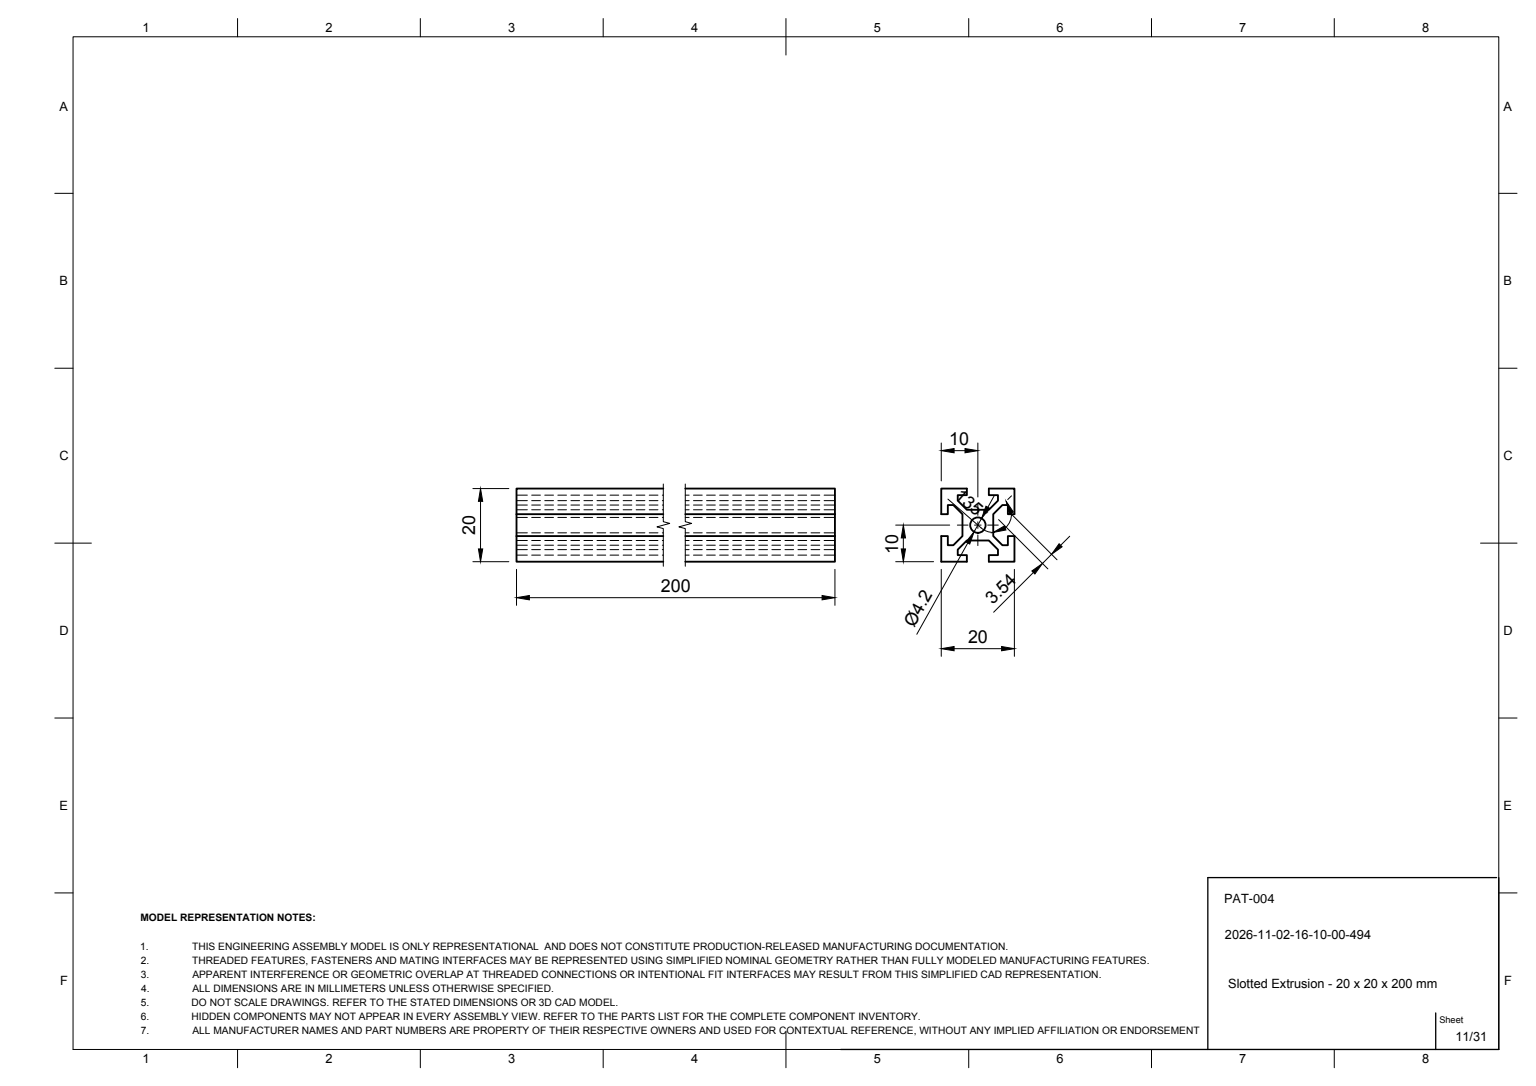
ISO-10303-21;
HEADER;
/* Generated by software containing ST-Developer
 * from STEP Tools, Inc. (www.steptools.com) 
 */

FILE_DESCRIPTION(
/* description */ ('Air blow-off nozzle station'),
/* implementation_level */ '2;1');

FILE_NAME(
/* name */ 'Slotted Extrusion - 20 x 20 x 200 mm.step',
/* time_stamp */ '2026-10-27T10:53:54-07:00',
/* author */ (''),
/* organization */ (''),
/* preprocessor_version */ 'ST-DEVELOPER v20.2',
/* originating_system */ 'Autodesk Translation Framework v15.17.0.0',
/* authorisation */ '');

FILE_SCHEMA (('AUTOMOTIVE_DESIGN { 1 0 10303 214 3 1 1 }'));
ENDSEC;

DATA;
#10=MECHANICAL_DESIGN_GEOMETRIC_PRESENTATION_REPRESENTATION('',(#246),#7897);
#196=SHAPE_REPRESENTATION_RELATIONSHIP('SRR','None',#8010,#221);
#221=ADVANCED_BREP_SHAPE_REPRESENTATION('',(#271),#7877);
#246=STYLED_ITEM('',(#8234),#271);
#271=MANIFOLD_SOLID_BREP('Body1',#4295);
#325=FACE_BOUND('',#967,.T.);
#326=FACE_BOUND('',#969,.T.);
#424=PLANE('',#4750);
#425=PLANE('',#4751);
#426=PLANE('',#4752);
#427=PLANE('',#4753);
#428=PLANE('',#4754);
#429=PLANE('',#4755);
#430=PLANE('',#4756);
#431=PLANE('',#4757);
#432=PLANE('',#4758);
#433=PLANE('',#4759);
#434=PLANE('',#4760);
#435=PLANE('',#4761);
#436=PLANE('',#4762);
#437=PLANE('',#4763);
#438=PLANE('',#4764);
#439=PLANE('',#4765);
#440=PLANE('',#4766);
#441=PLANE('',#4767);
#442=PLANE('',#4768);
#443=PLANE('',#4769);
#444=PLANE('',#4770);
#445=PLANE('',#4771);
#446=PLANE('',#4772);
#447=PLANE('',#4773);
#448=PLANE('',#4774);
#449=PLANE('',#4775);
#450=PLANE('',#4776);
#451=PLANE('',#4777);
#452=PLANE('',#4778);
#453=PLANE('',#4779);
#454=PLANE('',#4780);
#455=PLANE('',#4781);
#456=PLANE('',#4782);
#457=PLANE('',#4783);
#458=PLANE('',#4784);
#459=PLANE('',#4785);
#460=PLANE('',#4789);
#461=PLANE('',#4790);
#462=PLANE('',#4791);
#463=PLANE('',#4792);
#464=PLANE('',#4793);
#465=PLANE('',#4794);
#466=PLANE('',#4795);
#467=PLANE('',#4796);
#468=PLANE('',#4797);
#469=PLANE('',#4798);
#625=FACE_OUTER_BOUND('',#921,.T.);
#626=FACE_OUTER_BOUND('',#922,.T.);
#627=FACE_OUTER_BOUND('',#923,.T.);
#628=FACE_OUTER_BOUND('',#924,.T.);
#629=FACE_OUTER_BOUND('',#925,.T.);
#630=FACE_OUTER_BOUND('',#926,.T.);
#631=FACE_OUTER_BOUND('',#927,.T.);
#632=FACE_OUTER_BOUND('',#928,.T.);
#633=FACE_OUTER_BOUND('',#929,.T.);
#634=FACE_OUTER_BOUND('',#930,.T.);
#635=FACE_OUTER_BOUND('',#931,.T.);
#636=FACE_OUTER_BOUND('',#932,.T.);
#637=FACE_OUTER_BOUND('',#933,.T.);
#638=FACE_OUTER_BOUND('',#934,.T.);
#639=FACE_OUTER_BOUND('',#935,.T.);
#640=FACE_OUTER_BOUND('',#936,.T.);
#641=FACE_OUTER_BOUND('',#937,.T.);
#642=FACE_OUTER_BOUND('',#938,.T.);
#643=FACE_OUTER_BOUND('',#939,.T.);
#644=FACE_OUTER_BOUND('',#940,.T.);
#645=FACE_OUTER_BOUND('',#941,.T.);
#646=FACE_OUTER_BOUND('',#942,.T.);
#647=FACE_OUTER_BOUND('',#943,.T.);
#648=FACE_OUTER_BOUND('',#944,.T.);
#649=FACE_OUTER_BOUND('',#945,.T.);
#650=FACE_OUTER_BOUND('',#946,.T.);
#651=FACE_OUTER_BOUND('',#947,.T.);
#652=FACE_OUTER_BOUND('',#948,.T.);
#653=FACE_OUTER_BOUND('',#949,.T.);
#654=FACE_OUTER_BOUND('',#950,.T.);
#655=FACE_OUTER_BOUND('',#951,.T.);
#656=FACE_OUTER_BOUND('',#952,.T.);
#657=FACE_OUTER_BOUND('',#953,.T.);
#658=FACE_OUTER_BOUND('',#954,.T.);
#659=FACE_OUTER_BOUND('',#955,.T.);
#660=FACE_OUTER_BOUND('',#956,.T.);
#661=FACE_OUTER_BOUND('',#957,.T.);
#662=FACE_OUTER_BOUND('',#958,.T.);
#663=FACE_OUTER_BOUND('',#959,.T.);
#664=FACE_OUTER_BOUND('',#960,.T.);
#665=FACE_OUTER_BOUND('',#961,.T.);
#666=FACE_OUTER_BOUND('',#962,.T.);
#667=FACE_OUTER_BOUND('',#963,.T.);
#668=FACE_OUTER_BOUND('',#964,.T.);
#669=FACE_OUTER_BOUND('',#965,.T.);
#670=FACE_OUTER_BOUND('',#966,.T.);
#671=FACE_OUTER_BOUND('',#968,.T.);
#921=EDGE_LOOP('',(#3253,#3254,#3255,#3256));
#922=EDGE_LOOP('',(#3257,#3258,#3259,#3260));
#923=EDGE_LOOP('',(#3261,#3262,#3263,#3264));
#924=EDGE_LOOP('',(#3265,#3266,#3267,#3268));
#925=EDGE_LOOP('',(#3269,#3270,#3271,#3272));
#926=EDGE_LOOP('',(#3273,#3274,#3275,#3276));
#927=EDGE_LOOP('',(#3277,#3278,#3279,#3280));
#928=EDGE_LOOP('',(#3281,#3282,#3283,#3284));
#929=EDGE_LOOP('',(#3285,#3286,#3287,#3288));
#930=EDGE_LOOP('',(#3289,#3290,#3291,#3292));
#931=EDGE_LOOP('',(#3293,#3294,#3295,#3296));
#932=EDGE_LOOP('',(#3297,#3298,#3299,#3300));
#933=EDGE_LOOP('',(#3301,#3302,#3303,#3304));
#934=EDGE_LOOP('',(#3305,#3306,#3307,#3308));
#935=EDGE_LOOP('',(#3309,#3310,#3311,#3312));
#936=EDGE_LOOP('',(#3313,#3314,#3315,#3316));
#937=EDGE_LOOP('',(#3317,#3318,#3319,#3320));
#938=EDGE_LOOP('',(#3321,#3322,#3323,#3324));
#939=EDGE_LOOP('',(#3325,#3326,#3327,#3328));
#940=EDGE_LOOP('',(#3329,#3330,#3331,#3332));
#941=EDGE_LOOP('',(#3333,#3334,#3335,#3336));
#942=EDGE_LOOP('',(#3337,#3338,#3339,#3340));
#943=EDGE_LOOP('',(#3341,#3342,#3343,#3344));
#944=EDGE_LOOP('',(#3345,#3346,#3347,#3348));
#945=EDGE_LOOP('',(#3349,#3350,#3351,#3352));
#946=EDGE_LOOP('',(#3353,#3354,#3355,#3356));
#947=EDGE_LOOP('',(#3357,#3358,#3359,#3360));
#948=EDGE_LOOP('',(#3361,#3362,#3363,#3364));
#949=EDGE_LOOP('',(#3365,#3366,#3367,#3368));
#950=EDGE_LOOP('',(#3369,#3370,#3371,#3372));
#951=EDGE_LOOP('',(#3373,#3374,#3375,#3376));
#952=EDGE_LOOP('',(#3377,#3378,#3379,#3380));
#953=EDGE_LOOP('',(#3381,#3382,#3383,#3384));
#954=EDGE_LOOP('',(#3385,#3386,#3387,#3388));
#955=EDGE_LOOP('',(#3389,#3390,#3391,#3392));
#956=EDGE_LOOP('',(#3393,#3394,#3395,#3396));
#957=EDGE_LOOP('',(#3397,#3398,#3399,#3400));
#958=EDGE_LOOP('',(#3401,#3402,#3403,#3404));
#959=EDGE_LOOP('',(#3405,#3406,#3407,#3408));
#960=EDGE_LOOP('',(#3409,#3410,#3411,#3412));
#961=EDGE_LOOP('',(#3413,#3414,#3415,#3416));
#962=EDGE_LOOP('',(#3417,#3418,#3419,#3420));
#963=EDGE_LOOP('',(#3421,#3422,#3423,#3424));
#964=EDGE_LOOP('',(#3425,#3426,#3427,#3428));
#965=EDGE_LOOP('',(#3429,#3430,#3431,#3432));
#966=EDGE_LOOP('',(#3433,#3434,#3435,#3436,#3437,#3438,#3439,#3440,#3441,
#3442,#3443,#3444,#3445,#3446,#3447,#3448,#3449,#3450,#3451,#3452,#3453,
#3454,#3455,#3456,#3457,#3458,#3459,#3460,#3461,#3462,#3463,#3464,#3465,
#3466,#3467,#3468,#3469,#3470,#3471,#3472,#3473,#3474,#3475,#3476));
#967=EDGE_LOOP('',(#3477));
#968=EDGE_LOOP('',(#3478,#3479,#3480,#3481,#3482,#3483,#3484,#3485,#3486,
#3487,#3488,#3489,#3490,#3491,#3492,#3493,#3494,#3495,#3496,#3497,#3498,
#3499,#3500,#3501,#3502,#3503,#3504,#3505,#3506,#3507,#3508,#3509,#3510,
#3511,#3512,#3513,#3514,#3515,#3516,#3517,#3518,#3519,#3520,#3521));
#969=EDGE_LOOP('',(#3522));
#1236=LINE('',#7023,#1590);
#1237=LINE('',#7025,#1591);
#1238=LINE('',#7027,#1592);
#1239=LINE('',#7028,#1593);
#1240=LINE('',#7031,#1594);
#1241=LINE('',#7033,#1595);
#1242=LINE('',#7034,#1596);
#1243=LINE('',#7037,#1597);
#1244=LINE('',#7039,#1598);
#1245=LINE('',#7040,#1599);
#1246=LINE('',#7043,#1600);
#1247=LINE('',#7045,#1601);
#1248=LINE('',#7046,#1602);
#1249=LINE('',#7049,#1603);
#1250=LINE('',#7051,#1604);
#1251=LINE('',#7052,#1605);
#1252=LINE('',#7055,#1606);
#1253=LINE('',#7057,#1607);
#1254=LINE('',#7058,#1608);
#1255=LINE('',#7061,#1609);
#1256=LINE('',#7063,#1610);
#1257=LINE('',#7064,#1611);
#1258=LINE('',#7067,#1612);
#1259=LINE('',#7069,#1613);
#1260=LINE('',#7070,#1614);
#1261=LINE('',#7073,#1615);
#1262=LINE('',#7075,#1616);
#1263=LINE('',#7076,#1617);
#1264=LINE('',#7080,#1618);
#1265=LINE('',#7082,#1619);
#1266=LINE('',#7084,#1620);
#1267=LINE('',#7085,#1621);
#1268=LINE('',#7088,#1622);
#1269=LINE('',#7090,#1623);
#1270=LINE('',#7091,#1624);
#1271=LINE('',#7094,#1625);
#1272=LINE('',#7096,#1626);
#1273=LINE('',#7097,#1627);
#1274=LINE('',#7100,#1628);
#1275=LINE('',#7102,#1629);
#1276=LINE('',#7103,#1630);
#1277=LINE('',#7106,#1631);
#1278=LINE('',#7108,#1632);
#1279=LINE('',#7109,#1633);
#1280=LINE('',#7112,#1634);
#1281=LINE('',#7114,#1635);
#1282=LINE('',#7115,#1636);
#1283=LINE('',#7118,#1637);
#1284=LINE('',#7120,#1638);
#1285=LINE('',#7121,#1639);
#1286=LINE('',#7124,#1640);
#1287=LINE('',#7126,#1641);
#1288=LINE('',#7127,#1642);
#1289=LINE('',#7130,#1643);
#1290=LINE('',#7132,#1644);
#1291=LINE('',#7133,#1645);
#1292=LINE('',#7137,#1646);
#1293=LINE('',#7139,#1647);
#1294=LINE('',#7141,#1648);
#1295=LINE('',#7142,#1649);
#1296=LINE('',#7145,#1650);
#1297=LINE('',#7147,#1651);
#1298=LINE('',#7148,#1652);
#1299=LINE('',#7151,#1653);
#1300=LINE('',#7153,#1654);
#1301=LINE('',#7154,#1655);
#1302=LINE('',#7157,#1656);
#1303=LINE('',#7159,#1657);
#1304=LINE('',#7160,#1658);
#1305=LINE('',#7163,#1659);
#1306=LINE('',#7165,#1660);
#1307=LINE('',#7166,#1661);
#1308=LINE('',#7169,#1662);
#1309=LINE('',#7171,#1663);
#1310=LINE('',#7172,#1664);
#1311=LINE('',#7175,#1665);
#1312=LINE('',#7177,#1666);
#1313=LINE('',#7178,#1667);
#1314=LINE('',#7181,#1668);
#1315=LINE('',#7183,#1669);
#1316=LINE('',#7184,#1670);
#1317=LINE('',#7187,#1671);
#1318=LINE('',#7189,#1672);
#1319=LINE('',#7190,#1673);
#1320=LINE('',#7194,#1674);
#1321=LINE('',#7196,#1675);
#1322=LINE('',#7198,#1676);
#1323=LINE('',#7199,#1677);
#1324=LINE('',#7202,#1678);
#1325=LINE('',#7204,#1679);
#1326=LINE('',#7205,#1680);
#1327=LINE('',#7208,#1681);
#1328=LINE('',#7210,#1682);
#1329=LINE('',#7211,#1683);
#1330=LINE('',#7214,#1684);
#1331=LINE('',#7216,#1685);
#1332=LINE('',#7217,#1686);
#1333=LINE('',#7220,#1687);
#1334=LINE('',#7222,#1688);
#1335=LINE('',#7223,#1689);
#1336=LINE('',#7226,#1690);
#1337=LINE('',#7228,#1691);
#1338=LINE('',#7229,#1692);
#1339=LINE('',#7232,#1693);
#1340=LINE('',#7234,#1694);
#1341=LINE('',#7235,#1695);
#1342=LINE('',#7238,#1696);
#1343=LINE('',#7240,#1697);
#1344=LINE('',#7241,#1698);
#1345=LINE('',#7244,#1699);
#1346=LINE('',#7246,#1700);
#1347=LINE('',#7247,#1701);
#1348=LINE('',#7252,#1702);
#1349=LINE('',#7256,#1703);
#1350=LINE('',#7258,#1704);
#1351=LINE('',#7259,#1705);
#1352=LINE('',#7262,#1706);
#1353=LINE('',#7264,#1707);
#1354=LINE('',#7265,#1708);
#1355=LINE('',#7267,#1709);
#1356=LINE('',#7268,#1710);
#1357=LINE('',#7271,#1711);
#1358=LINE('',#7273,#1712);
#1359=LINE('',#7274,#1713);
#1360=LINE('',#7276,#1714);
#1361=LINE('',#7277,#1715);
#1362=LINE('',#7280,#1716);
#1363=LINE('',#7282,#1717);
#1364=LINE('',#7283,#1718);
#1365=LINE('',#7285,#1719);
#1366=LINE('',#7286,#1720);
#1367=LINE('',#7288,#1721);
#1368=LINE('',#7289,#1722);
#1590=VECTOR('',#5494,1.);
#1591=VECTOR('',#5495,1.);
#1592=VECTOR('',#5496,1.);
#1593=VECTOR('',#5497,1.);
#1594=VECTOR('',#5500,1.);
#1595=VECTOR('',#5501,1.);
#1596=VECTOR('',#5502,1.);
#1597=VECTOR('',#5505,1.);
#1598=VECTOR('',#5506,1.);
#1599=VECTOR('',#5507,1.);
#1600=VECTOR('',#5510,1.);
#1601=VECTOR('',#5511,1.);
#1602=VECTOR('',#5512,1.);
#1603=VECTOR('',#5515,1.);
#1604=VECTOR('',#5516,1.);
#1605=VECTOR('',#5517,1.);
#1606=VECTOR('',#5520,1.);
#1607=VECTOR('',#5521,1.);
#1608=VECTOR('',#5522,1.);
#1609=VECTOR('',#5525,1.);
#1610=VECTOR('',#5526,1.);
#1611=VECTOR('',#5527,1.);
#1612=VECTOR('',#5530,1.);
#1613=VECTOR('',#5531,1.);
#1614=VECTOR('',#5532,1.);
#1615=VECTOR('',#5535,1.);
#1616=VECTOR('',#5536,1.);
#1617=VECTOR('',#5537,1.);
#1618=VECTOR('',#5540,1.);
#1619=VECTOR('',#5541,1.);
#1620=VECTOR('',#5542,1.);
#1621=VECTOR('',#5543,1.);
#1622=VECTOR('',#5546,1.);
#1623=VECTOR('',#5547,1.);
#1624=VECTOR('',#5548,1.);
#1625=VECTOR('',#5551,1.);
#1626=VECTOR('',#5552,1.);
#1627=VECTOR('',#5553,1.);
#1628=VECTOR('',#5556,1.);
#1629=VECTOR('',#5557,1.);
#1630=VECTOR('',#5558,1.);
#1631=VECTOR('',#5561,1.);
#1632=VECTOR('',#5562,1.);
#1633=VECTOR('',#5563,1.);
#1634=VECTOR('',#5566,1.);
#1635=VECTOR('',#5567,1.);
#1636=VECTOR('',#5568,1.);
#1637=VECTOR('',#5571,1.);
#1638=VECTOR('',#5572,1.);
#1639=VECTOR('',#5573,1.);
#1640=VECTOR('',#5576,1.);
#1641=VECTOR('',#5577,1.);
#1642=VECTOR('',#5578,1.);
#1643=VECTOR('',#5581,1.);
#1644=VECTOR('',#5582,1.);
#1645=VECTOR('',#5583,1.);
#1646=VECTOR('',#5586,1.);
#1647=VECTOR('',#5587,1.);
#1648=VECTOR('',#5588,1.);
#1649=VECTOR('',#5589,1.);
#1650=VECTOR('',#5592,1.);
#1651=VECTOR('',#5593,1.);
#1652=VECTOR('',#5594,1.);
#1653=VECTOR('',#5597,1.);
#1654=VECTOR('',#5598,1.);
#1655=VECTOR('',#5599,1.);
#1656=VECTOR('',#5602,1.);
#1657=VECTOR('',#5603,1.);
#1658=VECTOR('',#5604,1.);
#1659=VECTOR('',#5607,1.);
#1660=VECTOR('',#5608,1.);
#1661=VECTOR('',#5609,1.);
#1662=VECTOR('',#5612,1.);
#1663=VECTOR('',#5613,1.);
#1664=VECTOR('',#5614,1.);
#1665=VECTOR('',#5617,1.);
#1666=VECTOR('',#5618,1.);
#1667=VECTOR('',#5619,1.);
#1668=VECTOR('',#5622,1.);
#1669=VECTOR('',#5623,1.);
#1670=VECTOR('',#5624,1.);
#1671=VECTOR('',#5627,1.);
#1672=VECTOR('',#5628,1.);
#1673=VECTOR('',#5629,1.);
#1674=VECTOR('',#5632,1.);
#1675=VECTOR('',#5633,1.);
#1676=VECTOR('',#5634,1.);
#1677=VECTOR('',#5635,1.);
#1678=VECTOR('',#5638,1.);
#1679=VECTOR('',#5639,1.);
#1680=VECTOR('',#5640,1.);
#1681=VECTOR('',#5643,1.);
#1682=VECTOR('',#5644,1.);
#1683=VECTOR('',#5645,1.);
#1684=VECTOR('',#5648,1.);
#1685=VECTOR('',#5649,1.);
#1686=VECTOR('',#5650,1.);
#1687=VECTOR('',#5653,1.);
#1688=VECTOR('',#5654,1.);
#1689=VECTOR('',#5655,1.);
#1690=VECTOR('',#5658,1.);
#1691=VECTOR('',#5659,1.);
#1692=VECTOR('',#5660,1.);
#1693=VECTOR('',#5663,1.);
#1694=VECTOR('',#5664,1.);
#1695=VECTOR('',#5665,1.);
#1696=VECTOR('',#5668,1.);
#1697=VECTOR('',#5669,1.);
#1698=VECTOR('',#5670,1.);
#1699=VECTOR('',#5673,1.);
#1700=VECTOR('',#5674,1.);
#1701=VECTOR('',#5675,1.);
#1702=VECTOR('',#5680,0.21);
#1703=VECTOR('',#5685,1.);
#1704=VECTOR('',#5686,1.);
#1705=VECTOR('',#5687,1.);
#1706=VECTOR('',#5690,1.);
#1707=VECTOR('',#5691,1.);
#1708=VECTOR('',#5692,1.);
#1709=VECTOR('',#5695,1.);
#1710=VECTOR('',#5696,1.);
#1711=VECTOR('',#5699,1.);
#1712=VECTOR('',#5700,1.);
#1713=VECTOR('',#5701,1.);
#1714=VECTOR('',#5704,1.);
#1715=VECTOR('',#5705,1.);
#1716=VECTOR('',#5708,1.);
#1717=VECTOR('',#5709,1.);
#1718=VECTOR('',#5710,1.);
#1719=VECTOR('',#5713,1.);
#1720=VECTOR('',#5714,1.);
#1721=VECTOR('',#5717,1.);
#1722=VECTOR('',#5718,1.);
#1910=CIRCLE('',#4787,0.21);
#1911=CIRCLE('',#4788,0.21);
#2130=VERTEX_POINT('',#7021);
#2131=VERTEX_POINT('',#7022);
#2132=VERTEX_POINT('',#7024);
#2133=VERTEX_POINT('',#7026);
#2134=VERTEX_POINT('',#7030);
#2135=VERTEX_POINT('',#7032);
#2136=VERTEX_POINT('',#7036);
#2137=VERTEX_POINT('',#7038);
#2138=VERTEX_POINT('',#7042);
#2139=VERTEX_POINT('',#7044);
#2140=VERTEX_POINT('',#7048);
#2141=VERTEX_POINT('',#7050);
#2142=VERTEX_POINT('',#7054);
#2143=VERTEX_POINT('',#7056);
#2144=VERTEX_POINT('',#7060);
#2145=VERTEX_POINT('',#7062);
#2146=VERTEX_POINT('',#7066);
#2147=VERTEX_POINT('',#7068);
#2148=VERTEX_POINT('',#7072);
#2149=VERTEX_POINT('',#7074);
#2150=VERTEX_POINT('',#7078);
#2151=VERTEX_POINT('',#7079);
#2152=VERTEX_POINT('',#7081);
#2153=VERTEX_POINT('',#7083);
#2154=VERTEX_POINT('',#7087);
#2155=VERTEX_POINT('',#7089);
#2156=VERTEX_POINT('',#7093);
#2157=VERTEX_POINT('',#7095);
#2158=VERTEX_POINT('',#7099);
#2159=VERTEX_POINT('',#7101);
#2160=VERTEX_POINT('',#7105);
#2161=VERTEX_POINT('',#7107);
#2162=VERTEX_POINT('',#7111);
#2163=VERTEX_POINT('',#7113);
#2164=VERTEX_POINT('',#7117);
#2165=VERTEX_POINT('',#7119);
#2166=VERTEX_POINT('',#7123);
#2167=VERTEX_POINT('',#7125);
#2168=VERTEX_POINT('',#7129);
#2169=VERTEX_POINT('',#7131);
#2170=VERTEX_POINT('',#7135);
#2171=VERTEX_POINT('',#7136);
#2172=VERTEX_POINT('',#7138);
#2173=VERTEX_POINT('',#7140);
#2174=VERTEX_POINT('',#7144);
#2175=VERTEX_POINT('',#7146);
#2176=VERTEX_POINT('',#7150);
#2177=VERTEX_POINT('',#7152);
#2178=VERTEX_POINT('',#7156);
#2179=VERTEX_POINT('',#7158);
#2180=VERTEX_POINT('',#7162);
#2181=VERTEX_POINT('',#7164);
#2182=VERTEX_POINT('',#7168);
#2183=VERTEX_POINT('',#7170);
#2184=VERTEX_POINT('',#7174);
#2185=VERTEX_POINT('',#7176);
#2186=VERTEX_POINT('',#7180);
#2187=VERTEX_POINT('',#7182);
#2188=VERTEX_POINT('',#7186);
#2189=VERTEX_POINT('',#7188);
#2190=VERTEX_POINT('',#7192);
#2191=VERTEX_POINT('',#7193);
#2192=VERTEX_POINT('',#7195);
#2193=VERTEX_POINT('',#7197);
#2194=VERTEX_POINT('',#7201);
#2195=VERTEX_POINT('',#7203);
#2196=VERTEX_POINT('',#7207);
#2197=VERTEX_POINT('',#7209);
#2198=VERTEX_POINT('',#7213);
#2199=VERTEX_POINT('',#7215);
#2200=VERTEX_POINT('',#7219);
#2201=VERTEX_POINT('',#7221);
#2202=VERTEX_POINT('',#7225);
#2203=VERTEX_POINT('',#7227);
#2204=VERTEX_POINT('',#7231);
#2205=VERTEX_POINT('',#7233);
#2206=VERTEX_POINT('',#7237);
#2207=VERTEX_POINT('',#7239);
#2208=VERTEX_POINT('',#7243);
#2209=VERTEX_POINT('',#7245);
#2210=VERTEX_POINT('',#7249);
#2211=VERTEX_POINT('',#7251);
#2212=VERTEX_POINT('',#7255);
#2213=VERTEX_POINT('',#7257);
#2214=VERTEX_POINT('',#7261);
#2215=VERTEX_POINT('',#7263);
#2216=VERTEX_POINT('',#7270);
#2217=VERTEX_POINT('',#7272);
#2218=VERTEX_POINT('',#7279);
#2219=VERTEX_POINT('',#7281);
#2544=EDGE_CURVE('',#2130,#2131,#1236,.T.);
#2545=EDGE_CURVE('',#2130,#2132,#1237,.T.);
#2546=EDGE_CURVE('',#2133,#2132,#1238,.T.);
#2547=EDGE_CURVE('',#2131,#2133,#1239,.T.);
#2548=EDGE_CURVE('',#2134,#2130,#1240,.T.);
#2549=EDGE_CURVE('',#2134,#2135,#1241,.T.);
#2550=EDGE_CURVE('',#2132,#2135,#1242,.T.);
#2551=EDGE_CURVE('',#2136,#2134,#1243,.T.);
#2552=EDGE_CURVE('',#2136,#2137,#1244,.T.);
#2553=EDGE_CURVE('',#2135,#2137,#1245,.T.);
#2554=EDGE_CURVE('',#2138,#2136,#1246,.T.);
#2555=EDGE_CURVE('',#2138,#2139,#1247,.T.);
#2556=EDGE_CURVE('',#2137,#2139,#1248,.T.);
#2557=EDGE_CURVE('',#2140,#2138,#1249,.T.);
#2558=EDGE_CURVE('',#2140,#2141,#1250,.T.);
#2559=EDGE_CURVE('',#2139,#2141,#1251,.T.);
#2560=EDGE_CURVE('',#2142,#2140,#1252,.T.);
#2561=EDGE_CURVE('',#2142,#2143,#1253,.T.);
#2562=EDGE_CURVE('',#2141,#2143,#1254,.T.);
#2563=EDGE_CURVE('',#2144,#2142,#1255,.T.);
#2564=EDGE_CURVE('',#2144,#2145,#1256,.T.);
#2565=EDGE_CURVE('',#2143,#2145,#1257,.T.);
#2566=EDGE_CURVE('',#2146,#2144,#1258,.T.);
#2567=EDGE_CURVE('',#2146,#2147,#1259,.T.);
#2568=EDGE_CURVE('',#2145,#2147,#1260,.T.);
#2569=EDGE_CURVE('',#2148,#2146,#1261,.T.);
#2570=EDGE_CURVE('',#2149,#2148,#1262,.T.);
#2571=EDGE_CURVE('',#2147,#2149,#1263,.T.);
#2572=EDGE_CURVE('',#2150,#2151,#1264,.T.);
#2573=EDGE_CURVE('',#2150,#2152,#1265,.T.);
#2574=EDGE_CURVE('',#2153,#2152,#1266,.T.);
#2575=EDGE_CURVE('',#2151,#2153,#1267,.T.);
#2576=EDGE_CURVE('',#2154,#2150,#1268,.T.);
#2577=EDGE_CURVE('',#2154,#2155,#1269,.T.);
#2578=EDGE_CURVE('',#2152,#2155,#1270,.T.);
#2579=EDGE_CURVE('',#2156,#2154,#1271,.T.);
#2580=EDGE_CURVE('',#2156,#2157,#1272,.T.);
#2581=EDGE_CURVE('',#2155,#2157,#1273,.T.);
#2582=EDGE_CURVE('',#2158,#2156,#1274,.T.);
#2583=EDGE_CURVE('',#2158,#2159,#1275,.T.);
#2584=EDGE_CURVE('',#2157,#2159,#1276,.T.);
#2585=EDGE_CURVE('',#2160,#2158,#1277,.T.);
#2586=EDGE_CURVE('',#2160,#2161,#1278,.T.);
#2587=EDGE_CURVE('',#2159,#2161,#1279,.T.);
#2588=EDGE_CURVE('',#2162,#2160,#1280,.T.);
#2589=EDGE_CURVE('',#2162,#2163,#1281,.T.);
#2590=EDGE_CURVE('',#2161,#2163,#1282,.T.);
#2591=EDGE_CURVE('',#2164,#2162,#1283,.T.);
#2592=EDGE_CURVE('',#2164,#2165,#1284,.T.);
#2593=EDGE_CURVE('',#2163,#2165,#1285,.T.);
#2594=EDGE_CURVE('',#2166,#2164,#1286,.T.);
#2595=EDGE_CURVE('',#2166,#2167,#1287,.T.);
#2596=EDGE_CURVE('',#2165,#2167,#1288,.T.);
#2597=EDGE_CURVE('',#2168,#2166,#1289,.T.);
#2598=EDGE_CURVE('',#2169,#2168,#1290,.T.);
#2599=EDGE_CURVE('',#2167,#2169,#1291,.T.);
#2600=EDGE_CURVE('',#2170,#2171,#1292,.T.);
#2601=EDGE_CURVE('',#2170,#2172,#1293,.T.);
#2602=EDGE_CURVE('',#2173,#2172,#1294,.T.);
#2603=EDGE_CURVE('',#2171,#2173,#1295,.T.);
#2604=EDGE_CURVE('',#2174,#2170,#1296,.T.);
#2605=EDGE_CURVE('',#2174,#2175,#1297,.T.);
#2606=EDGE_CURVE('',#2172,#2175,#1298,.T.);
#2607=EDGE_CURVE('',#2176,#2174,#1299,.T.);
#2608=EDGE_CURVE('',#2176,#2177,#1300,.T.);
#2609=EDGE_CURVE('',#2175,#2177,#1301,.T.);
#2610=EDGE_CURVE('',#2178,#2176,#1302,.T.);
#2611=EDGE_CURVE('',#2178,#2179,#1303,.T.);
#2612=EDGE_CURVE('',#2177,#2179,#1304,.T.);
#2613=EDGE_CURVE('',#2180,#2178,#1305,.T.);
#2614=EDGE_CURVE('',#2180,#2181,#1306,.T.);
#2615=EDGE_CURVE('',#2179,#2181,#1307,.T.);
#2616=EDGE_CURVE('',#2182,#2180,#1308,.T.);
#2617=EDGE_CURVE('',#2182,#2183,#1309,.T.);
#2618=EDGE_CURVE('',#2181,#2183,#1310,.T.);
#2619=EDGE_CURVE('',#2184,#2182,#1311,.T.);
#2620=EDGE_CURVE('',#2184,#2185,#1312,.T.);
#2621=EDGE_CURVE('',#2183,#2185,#1313,.T.);
#2622=EDGE_CURVE('',#2186,#2184,#1314,.T.);
#2623=EDGE_CURVE('',#2186,#2187,#1315,.T.);
#2624=EDGE_CURVE('',#2185,#2187,#1316,.T.);
#2625=EDGE_CURVE('',#2188,#2186,#1317,.T.);
#2626=EDGE_CURVE('',#2189,#2188,#1318,.T.);
#2627=EDGE_CURVE('',#2187,#2189,#1319,.T.);
#2628=EDGE_CURVE('',#2190,#2191,#1320,.T.);
#2629=EDGE_CURVE('',#2190,#2192,#1321,.T.);
#2630=EDGE_CURVE('',#2193,#2192,#1322,.T.);
#2631=EDGE_CURVE('',#2191,#2193,#1323,.T.);
#2632=EDGE_CURVE('',#2194,#2190,#1324,.T.);
#2633=EDGE_CURVE('',#2194,#2195,#1325,.T.);
#2634=EDGE_CURVE('',#2192,#2195,#1326,.T.);
#2635=EDGE_CURVE('',#2196,#2194,#1327,.T.);
#2636=EDGE_CURVE('',#2196,#2197,#1328,.T.);
#2637=EDGE_CURVE('',#2195,#2197,#1329,.T.);
#2638=EDGE_CURVE('',#2198,#2196,#1330,.T.);
#2639=EDGE_CURVE('',#2198,#2199,#1331,.T.);
#2640=EDGE_CURVE('',#2197,#2199,#1332,.T.);
#2641=EDGE_CURVE('',#2200,#2198,#1333,.T.);
#2642=EDGE_CURVE('',#2200,#2201,#1334,.T.);
#2643=EDGE_CURVE('',#2199,#2201,#1335,.T.);
#2644=EDGE_CURVE('',#2202,#2200,#1336,.T.);
#2645=EDGE_CURVE('',#2202,#2203,#1337,.T.);
#2646=EDGE_CURVE('',#2201,#2203,#1338,.T.);
#2647=EDGE_CURVE('',#2204,#2202,#1339,.T.);
#2648=EDGE_CURVE('',#2204,#2205,#1340,.T.);
#2649=EDGE_CURVE('',#2203,#2205,#1341,.T.);
#2650=EDGE_CURVE('',#2206,#2204,#1342,.T.);
#2651=EDGE_CURVE('',#2206,#2207,#1343,.T.);
#2652=EDGE_CURVE('',#2205,#2207,#1344,.T.);
#2653=EDGE_CURVE('',#2208,#2206,#1345,.T.);
#2654=EDGE_CURVE('',#2209,#2208,#1346,.T.);
#2655=EDGE_CURVE('',#2207,#2209,#1347,.T.);
#2656=EDGE_CURVE('',#2210,#2210,#1910,.T.);
#2657=EDGE_CURVE('',#2210,#2211,#1348,.T.);
#2658=EDGE_CURVE('',#2211,#2211,#1911,.T.);
#2659=EDGE_CURVE('',#2148,#2212,#1349,.T.);
#2660=EDGE_CURVE('',#2212,#2213,#1350,.T.);
#2661=EDGE_CURVE('',#2149,#2213,#1351,.T.);
#2662=EDGE_CURVE('',#2214,#2133,#1352,.T.);
#2663=EDGE_CURVE('',#2215,#2214,#1353,.T.);
#2664=EDGE_CURVE('',#2215,#2131,#1354,.T.);
#2665=EDGE_CURVE('',#2168,#2215,#1355,.T.);
#2666=EDGE_CURVE('',#2169,#2214,#1356,.T.);
#2667=EDGE_CURVE('',#2216,#2153,#1357,.T.);
#2668=EDGE_CURVE('',#2217,#2216,#1358,.T.);
#2669=EDGE_CURVE('',#2217,#2151,#1359,.T.);
#2670=EDGE_CURVE('',#2188,#2217,#1360,.T.);
#2671=EDGE_CURVE('',#2189,#2216,#1361,.T.);
#2672=EDGE_CURVE('',#2218,#2173,#1362,.T.);
#2673=EDGE_CURVE('',#2219,#2218,#1363,.T.);
#2674=EDGE_CURVE('',#2219,#2171,#1364,.T.);
#2675=EDGE_CURVE('',#2208,#2219,#1365,.T.);
#2676=EDGE_CURVE('',#2209,#2218,#1366,.T.);
#2677=EDGE_CURVE('',#2213,#2193,#1367,.T.);
#2678=EDGE_CURVE('',#2212,#2191,#1368,.T.);
#3253=ORIENTED_EDGE('',*,*,#2544,.F.);
#3254=ORIENTED_EDGE('',*,*,#2545,.T.);
#3255=ORIENTED_EDGE('',*,*,#2546,.F.);
#3256=ORIENTED_EDGE('',*,*,#2547,.F.);
#3257=ORIENTED_EDGE('',*,*,#2548,.F.);
#3258=ORIENTED_EDGE('',*,*,#2549,.T.);
#3259=ORIENTED_EDGE('',*,*,#2550,.F.);
#3260=ORIENTED_EDGE('',*,*,#2545,.F.);
#3261=ORIENTED_EDGE('',*,*,#2551,.F.);
#3262=ORIENTED_EDGE('',*,*,#2552,.T.);
#3263=ORIENTED_EDGE('',*,*,#2553,.F.);
#3264=ORIENTED_EDGE('',*,*,#2549,.F.);
#3265=ORIENTED_EDGE('',*,*,#2554,.F.);
#3266=ORIENTED_EDGE('',*,*,#2555,.T.);
#3267=ORIENTED_EDGE('',*,*,#2556,.F.);
#3268=ORIENTED_EDGE('',*,*,#2552,.F.);
#3269=ORIENTED_EDGE('',*,*,#2557,.F.);
#3270=ORIENTED_EDGE('',*,*,#2558,.T.);
#3271=ORIENTED_EDGE('',*,*,#2559,.F.);
#3272=ORIENTED_EDGE('',*,*,#2555,.F.);
#3273=ORIENTED_EDGE('',*,*,#2560,.F.);
#3274=ORIENTED_EDGE('',*,*,#2561,.T.);
#3275=ORIENTED_EDGE('',*,*,#2562,.F.);
#3276=ORIENTED_EDGE('',*,*,#2558,.F.);
#3277=ORIENTED_EDGE('',*,*,#2563,.F.);
#3278=ORIENTED_EDGE('',*,*,#2564,.T.);
#3279=ORIENTED_EDGE('',*,*,#2565,.F.);
#3280=ORIENTED_EDGE('',*,*,#2561,.F.);
#3281=ORIENTED_EDGE('',*,*,#2566,.F.);
#3282=ORIENTED_EDGE('',*,*,#2567,.T.);
#3283=ORIENTED_EDGE('',*,*,#2568,.F.);
#3284=ORIENTED_EDGE('',*,*,#2564,.F.);
#3285=ORIENTED_EDGE('',*,*,#2569,.F.);
#3286=ORIENTED_EDGE('',*,*,#2570,.F.);
#3287=ORIENTED_EDGE('',*,*,#2571,.F.);
#3288=ORIENTED_EDGE('',*,*,#2567,.F.);
#3289=ORIENTED_EDGE('',*,*,#2572,.F.);
#3290=ORIENTED_EDGE('',*,*,#2573,.T.);
#3291=ORIENTED_EDGE('',*,*,#2574,.F.);
#3292=ORIENTED_EDGE('',*,*,#2575,.F.);
#3293=ORIENTED_EDGE('',*,*,#2576,.F.);
#3294=ORIENTED_EDGE('',*,*,#2577,.T.);
#3295=ORIENTED_EDGE('',*,*,#2578,.F.);
#3296=ORIENTED_EDGE('',*,*,#2573,.F.);
#3297=ORIENTED_EDGE('',*,*,#2579,.F.);
#3298=ORIENTED_EDGE('',*,*,#2580,.T.);
#3299=ORIENTED_EDGE('',*,*,#2581,.F.);
#3300=ORIENTED_EDGE('',*,*,#2577,.F.);
#3301=ORIENTED_EDGE('',*,*,#2582,.F.);
#3302=ORIENTED_EDGE('',*,*,#2583,.T.);
#3303=ORIENTED_EDGE('',*,*,#2584,.F.);
#3304=ORIENTED_EDGE('',*,*,#2580,.F.);
#3305=ORIENTED_EDGE('',*,*,#2585,.F.);
#3306=ORIENTED_EDGE('',*,*,#2586,.T.);
#3307=ORIENTED_EDGE('',*,*,#2587,.F.);
#3308=ORIENTED_EDGE('',*,*,#2583,.F.);
#3309=ORIENTED_EDGE('',*,*,#2588,.F.);
#3310=ORIENTED_EDGE('',*,*,#2589,.T.);
#3311=ORIENTED_EDGE('',*,*,#2590,.F.);
#3312=ORIENTED_EDGE('',*,*,#2586,.F.);
#3313=ORIENTED_EDGE('',*,*,#2591,.F.);
#3314=ORIENTED_EDGE('',*,*,#2592,.T.);
#3315=ORIENTED_EDGE('',*,*,#2593,.F.);
#3316=ORIENTED_EDGE('',*,*,#2589,.F.);
#3317=ORIENTED_EDGE('',*,*,#2594,.F.);
#3318=ORIENTED_EDGE('',*,*,#2595,.T.);
#3319=ORIENTED_EDGE('',*,*,#2596,.F.);
#3320=ORIENTED_EDGE('',*,*,#2592,.F.);
#3321=ORIENTED_EDGE('',*,*,#2597,.F.);
#3322=ORIENTED_EDGE('',*,*,#2598,.F.);
#3323=ORIENTED_EDGE('',*,*,#2599,.F.);
#3324=ORIENTED_EDGE('',*,*,#2595,.F.);
#3325=ORIENTED_EDGE('',*,*,#2600,.F.);
#3326=ORIENTED_EDGE('',*,*,#2601,.T.);
#3327=ORIENTED_EDGE('',*,*,#2602,.F.);
#3328=ORIENTED_EDGE('',*,*,#2603,.F.);
#3329=ORIENTED_EDGE('',*,*,#2604,.F.);
#3330=ORIENTED_EDGE('',*,*,#2605,.T.);
#3331=ORIENTED_EDGE('',*,*,#2606,.F.);
#3332=ORIENTED_EDGE('',*,*,#2601,.F.);
#3333=ORIENTED_EDGE('',*,*,#2607,.F.);
#3334=ORIENTED_EDGE('',*,*,#2608,.T.);
#3335=ORIENTED_EDGE('',*,*,#2609,.F.);
#3336=ORIENTED_EDGE('',*,*,#2605,.F.);
#3337=ORIENTED_EDGE('',*,*,#2610,.F.);
#3338=ORIENTED_EDGE('',*,*,#2611,.T.);
#3339=ORIENTED_EDGE('',*,*,#2612,.F.);
#3340=ORIENTED_EDGE('',*,*,#2608,.F.);
#3341=ORIENTED_EDGE('',*,*,#2613,.F.);
#3342=ORIENTED_EDGE('',*,*,#2614,.T.);
#3343=ORIENTED_EDGE('',*,*,#2615,.F.);
#3344=ORIENTED_EDGE('',*,*,#2611,.F.);
#3345=ORIENTED_EDGE('',*,*,#2616,.F.);
#3346=ORIENTED_EDGE('',*,*,#2617,.T.);
#3347=ORIENTED_EDGE('',*,*,#2618,.F.);
#3348=ORIENTED_EDGE('',*,*,#2614,.F.);
#3349=ORIENTED_EDGE('',*,*,#2619,.F.);
#3350=ORIENTED_EDGE('',*,*,#2620,.T.);
#3351=ORIENTED_EDGE('',*,*,#2621,.F.);
#3352=ORIENTED_EDGE('',*,*,#2617,.F.);
#3353=ORIENTED_EDGE('',*,*,#2622,.F.);
#3354=ORIENTED_EDGE('',*,*,#2623,.T.);
#3355=ORIENTED_EDGE('',*,*,#2624,.F.);
#3356=ORIENTED_EDGE('',*,*,#2620,.F.);
#3357=ORIENTED_EDGE('',*,*,#2625,.F.);
#3358=ORIENTED_EDGE('',*,*,#2626,.F.);
#3359=ORIENTED_EDGE('',*,*,#2627,.F.);
#3360=ORIENTED_EDGE('',*,*,#2623,.F.);
#3361=ORIENTED_EDGE('',*,*,#2628,.F.);
#3362=ORIENTED_EDGE('',*,*,#2629,.T.);
#3363=ORIENTED_EDGE('',*,*,#2630,.F.);
#3364=ORIENTED_EDGE('',*,*,#2631,.F.);
#3365=ORIENTED_EDGE('',*,*,#2632,.F.);
#3366=ORIENTED_EDGE('',*,*,#2633,.T.);
#3367=ORIENTED_EDGE('',*,*,#2634,.F.);
#3368=ORIENTED_EDGE('',*,*,#2629,.F.);
#3369=ORIENTED_EDGE('',*,*,#2635,.F.);
#3370=ORIENTED_EDGE('',*,*,#2636,.T.);
#3371=ORIENTED_EDGE('',*,*,#2637,.F.);
#3372=ORIENTED_EDGE('',*,*,#2633,.F.);
#3373=ORIENTED_EDGE('',*,*,#2638,.F.);
#3374=ORIENTED_EDGE('',*,*,#2639,.T.);
#3375=ORIENTED_EDGE('',*,*,#2640,.F.);
#3376=ORIENTED_EDGE('',*,*,#2636,.F.);
#3377=ORIENTED_EDGE('',*,*,#2641,.F.);
#3378=ORIENTED_EDGE('',*,*,#2642,.T.);
#3379=ORIENTED_EDGE('',*,*,#2643,.F.);
#3380=ORIENTED_EDGE('',*,*,#2639,.F.);
#3381=ORIENTED_EDGE('',*,*,#2644,.F.);
#3382=ORIENTED_EDGE('',*,*,#2645,.T.);
#3383=ORIENTED_EDGE('',*,*,#2646,.F.);
#3384=ORIENTED_EDGE('',*,*,#2642,.F.);
#3385=ORIENTED_EDGE('',*,*,#2647,.F.);
#3386=ORIENTED_EDGE('',*,*,#2648,.T.);
#3387=ORIENTED_EDGE('',*,*,#2649,.F.);
#3388=ORIENTED_EDGE('',*,*,#2645,.F.);
#3389=ORIENTED_EDGE('',*,*,#2650,.F.);
#3390=ORIENTED_EDGE('',*,*,#2651,.T.);
#3391=ORIENTED_EDGE('',*,*,#2652,.F.);
#3392=ORIENTED_EDGE('',*,*,#2648,.F.);
#3393=ORIENTED_EDGE('',*,*,#2653,.F.);
#3394=ORIENTED_EDGE('',*,*,#2654,.F.);
#3395=ORIENTED_EDGE('',*,*,#2655,.F.);
#3396=ORIENTED_EDGE('',*,*,#2651,.F.);
#3397=ORIENTED_EDGE('',*,*,#2656,.F.);
#3398=ORIENTED_EDGE('',*,*,#2657,.T.);
#3399=ORIENTED_EDGE('',*,*,#2658,.F.);
#3400=ORIENTED_EDGE('',*,*,#2657,.F.);
#3401=ORIENTED_EDGE('',*,*,#2570,.T.);
#3402=ORIENTED_EDGE('',*,*,#2659,.T.);
#3403=ORIENTED_EDGE('',*,*,#2660,.T.);
#3404=ORIENTED_EDGE('',*,*,#2661,.F.);
#3405=ORIENTED_EDGE('',*,*,#2547,.T.);
#3406=ORIENTED_EDGE('',*,*,#2662,.F.);
#3407=ORIENTED_EDGE('',*,*,#2663,.F.);
#3408=ORIENTED_EDGE('',*,*,#2664,.T.);
#3409=ORIENTED_EDGE('',*,*,#2598,.T.);
#3410=ORIENTED_EDGE('',*,*,#2665,.T.);
#3411=ORIENTED_EDGE('',*,*,#2663,.T.);
#3412=ORIENTED_EDGE('',*,*,#2666,.F.);
#3413=ORIENTED_EDGE('',*,*,#2575,.T.);
#3414=ORIENTED_EDGE('',*,*,#2667,.F.);
#3415=ORIENTED_EDGE('',*,*,#2668,.F.);
#3416=ORIENTED_EDGE('',*,*,#2669,.T.);
#3417=ORIENTED_EDGE('',*,*,#2626,.T.);
#3418=ORIENTED_EDGE('',*,*,#2670,.T.);
#3419=ORIENTED_EDGE('',*,*,#2668,.T.);
#3420=ORIENTED_EDGE('',*,*,#2671,.F.);
#3421=ORIENTED_EDGE('',*,*,#2603,.T.);
#3422=ORIENTED_EDGE('',*,*,#2672,.F.);
#3423=ORIENTED_EDGE('',*,*,#2673,.F.);
#3424=ORIENTED_EDGE('',*,*,#2674,.T.);
#3425=ORIENTED_EDGE('',*,*,#2654,.T.);
#3426=ORIENTED_EDGE('',*,*,#2675,.T.);
#3427=ORIENTED_EDGE('',*,*,#2673,.T.);
#3428=ORIENTED_EDGE('',*,*,#2676,.F.);
#3429=ORIENTED_EDGE('',*,*,#2631,.T.);
#3430=ORIENTED_EDGE('',*,*,#2677,.F.);
#3431=ORIENTED_EDGE('',*,*,#2660,.F.);
#3432=ORIENTED_EDGE('',*,*,#2678,.T.);
#3433=ORIENTED_EDGE('',*,*,#2546,.T.);
#3434=ORIENTED_EDGE('',*,*,#2550,.T.);
#3435=ORIENTED_EDGE('',*,*,#2553,.T.);
#3436=ORIENTED_EDGE('',*,*,#2556,.T.);
#3437=ORIENTED_EDGE('',*,*,#2559,.T.);
#3438=ORIENTED_EDGE('',*,*,#2562,.T.);
#3439=ORIENTED_EDGE('',*,*,#2565,.T.);
#3440=ORIENTED_EDGE('',*,*,#2568,.T.);
#3441=ORIENTED_EDGE('',*,*,#2571,.T.);
#3442=ORIENTED_EDGE('',*,*,#2661,.T.);
#3443=ORIENTED_EDGE('',*,*,#2677,.T.);
#3444=ORIENTED_EDGE('',*,*,#2630,.T.);
#3445=ORIENTED_EDGE('',*,*,#2634,.T.);
#3446=ORIENTED_EDGE('',*,*,#2637,.T.);
#3447=ORIENTED_EDGE('',*,*,#2640,.T.);
#3448=ORIENTED_EDGE('',*,*,#2643,.T.);
#3449=ORIENTED_EDGE('',*,*,#2646,.T.);
#3450=ORIENTED_EDGE('',*,*,#2649,.T.);
#3451=ORIENTED_EDGE('',*,*,#2652,.T.);
#3452=ORIENTED_EDGE('',*,*,#2655,.T.);
#3453=ORIENTED_EDGE('',*,*,#2676,.T.);
#3454=ORIENTED_EDGE('',*,*,#2672,.T.);
#3455=ORIENTED_EDGE('',*,*,#2602,.T.);
#3456=ORIENTED_EDGE('',*,*,#2606,.T.);
#3457=ORIENTED_EDGE('',*,*,#2609,.T.);
#3458=ORIENTED_EDGE('',*,*,#2612,.T.);
#3459=ORIENTED_EDGE('',*,*,#2615,.T.);
#3460=ORIENTED_EDGE('',*,*,#2618,.T.);
#3461=ORIENTED_EDGE('',*,*,#2621,.T.);
#3462=ORIENTED_EDGE('',*,*,#2624,.T.);
#3463=ORIENTED_EDGE('',*,*,#2627,.T.);
#3464=ORIENTED_EDGE('',*,*,#2671,.T.);
#3465=ORIENTED_EDGE('',*,*,#2667,.T.);
#3466=ORIENTED_EDGE('',*,*,#2574,.T.);
#3467=ORIENTED_EDGE('',*,*,#2578,.T.);
#3468=ORIENTED_EDGE('',*,*,#2581,.T.);
#3469=ORIENTED_EDGE('',*,*,#2584,.T.);
#3470=ORIENTED_EDGE('',*,*,#2587,.T.);
#3471=ORIENTED_EDGE('',*,*,#2590,.T.);
#3472=ORIENTED_EDGE('',*,*,#2593,.T.);
#3473=ORIENTED_EDGE('',*,*,#2596,.T.);
#3474=ORIENTED_EDGE('',*,*,#2599,.T.);
#3475=ORIENTED_EDGE('',*,*,#2666,.T.);
#3476=ORIENTED_EDGE('',*,*,#2662,.T.);
#3477=ORIENTED_EDGE('',*,*,#2658,.T.);
#3478=ORIENTED_EDGE('',*,*,#2544,.T.);
#3479=ORIENTED_EDGE('',*,*,#2664,.F.);
#3480=ORIENTED_EDGE('',*,*,#2665,.F.);
#3481=ORIENTED_EDGE('',*,*,#2597,.T.);
#3482=ORIENTED_EDGE('',*,*,#2594,.T.);
#3483=ORIENTED_EDGE('',*,*,#2591,.T.);
#3484=ORIENTED_EDGE('',*,*,#2588,.T.);
#3485=ORIENTED_EDGE('',*,*,#2585,.T.);
#3486=ORIENTED_EDGE('',*,*,#2582,.T.);
#3487=ORIENTED_EDGE('',*,*,#2579,.T.);
#3488=ORIENTED_EDGE('',*,*,#2576,.T.);
#3489=ORIENTED_EDGE('',*,*,#2572,.T.);
#3490=ORIENTED_EDGE('',*,*,#2669,.F.);
#3491=ORIENTED_EDGE('',*,*,#2670,.F.);
#3492=ORIENTED_EDGE('',*,*,#2625,.T.);
#3493=ORIENTED_EDGE('',*,*,#2622,.T.);
#3494=ORIENTED_EDGE('',*,*,#2619,.T.);
#3495=ORIENTED_EDGE('',*,*,#2616,.T.);
#3496=ORIENTED_EDGE('',*,*,#2613,.T.);
#3497=ORIENTED_EDGE('',*,*,#2610,.T.);
#3498=ORIENTED_EDGE('',*,*,#2607,.T.);
#3499=ORIENTED_EDGE('',*,*,#2604,.T.);
#3500=ORIENTED_EDGE('',*,*,#2600,.T.);
#3501=ORIENTED_EDGE('',*,*,#2674,.F.);
#3502=ORIENTED_EDGE('',*,*,#2675,.F.);
#3503=ORIENTED_EDGE('',*,*,#2653,.T.);
#3504=ORIENTED_EDGE('',*,*,#2650,.T.);
#3505=ORIENTED_EDGE('',*,*,#2647,.T.);
#3506=ORIENTED_EDGE('',*,*,#2644,.T.);
#3507=ORIENTED_EDGE('',*,*,#2641,.T.);
#3508=ORIENTED_EDGE('',*,*,#2638,.T.);
#3509=ORIENTED_EDGE('',*,*,#2635,.T.);
#3510=ORIENTED_EDGE('',*,*,#2632,.T.);
#3511=ORIENTED_EDGE('',*,*,#2628,.T.);
#3512=ORIENTED_EDGE('',*,*,#2678,.F.);
#3513=ORIENTED_EDGE('',*,*,#2659,.F.);
#3514=ORIENTED_EDGE('',*,*,#2569,.T.);
#3515=ORIENTED_EDGE('',*,*,#2566,.T.);
#3516=ORIENTED_EDGE('',*,*,#2563,.T.);
#3517=ORIENTED_EDGE('',*,*,#2560,.T.);
#3518=ORIENTED_EDGE('',*,*,#2557,.T.);
#3519=ORIENTED_EDGE('',*,*,#2554,.T.);
#3520=ORIENTED_EDGE('',*,*,#2551,.T.);
#3521=ORIENTED_EDGE('',*,*,#2548,.T.);
#3522=ORIENTED_EDGE('',*,*,#2656,.T.);
#3988=CYLINDRICAL_SURFACE('',#4786,0.21);
#4115=ADVANCED_FACE('',(#625),#424,.F.);
#4116=ADVANCED_FACE('',(#626),#425,.F.);
#4117=ADVANCED_FACE('',(#627),#426,.F.);
#4118=ADVANCED_FACE('',(#628),#427,.F.);
#4119=ADVANCED_FACE('',(#629),#428,.F.);
#4120=ADVANCED_FACE('',(#630),#429,.F.);
#4121=ADVANCED_FACE('',(#631),#430,.F.);
#4122=ADVANCED_FACE('',(#632),#431,.F.);
#4123=ADVANCED_FACE('',(#633),#432,.F.);
#4124=ADVANCED_FACE('',(#634),#433,.F.);
#4125=ADVANCED_FACE('',(#635),#434,.F.);
#4126=ADVANCED_FACE('',(#636),#435,.F.);
#4127=ADVANCED_FACE('',(#637),#436,.F.);
#4128=ADVANCED_FACE('',(#638),#437,.F.);
#4129=ADVANCED_FACE('',(#639),#438,.F.);
#4130=ADVANCED_FACE('',(#640),#439,.F.);
#4131=ADVANCED_FACE('',(#641),#440,.F.);
#4132=ADVANCED_FACE('',(#642),#441,.F.);
#4133=ADVANCED_FACE('',(#643),#442,.F.);
#4134=ADVANCED_FACE('',(#644),#443,.F.);
#4135=ADVANCED_FACE('',(#645),#444,.F.);
#4136=ADVANCED_FACE('',(#646),#445,.F.);
#4137=ADVANCED_FACE('',(#647),#446,.F.);
#4138=ADVANCED_FACE('',(#648),#447,.F.);
#4139=ADVANCED_FACE('',(#649),#448,.F.);
#4140=ADVANCED_FACE('',(#650),#449,.F.);
#4141=ADVANCED_FACE('',(#651),#450,.F.);
#4142=ADVANCED_FACE('',(#652),#451,.F.);
#4143=ADVANCED_FACE('',(#653),#452,.F.);
#4144=ADVANCED_FACE('',(#654),#453,.F.);
#4145=ADVANCED_FACE('',(#655),#454,.F.);
#4146=ADVANCED_FACE('',(#656),#455,.F.);
#4147=ADVANCED_FACE('',(#657),#456,.F.);
#4148=ADVANCED_FACE('',(#658),#457,.F.);
#4149=ADVANCED_FACE('',(#659),#458,.F.);
#4150=ADVANCED_FACE('',(#660),#459,.F.);
#4151=ADVANCED_FACE('',(#661),#3988,.F.);
#4152=ADVANCED_FACE('',(#662),#460,.T.);
#4153=ADVANCED_FACE('',(#663),#461,.T.);
#4154=ADVANCED_FACE('',(#664),#462,.T.);
#4155=ADVANCED_FACE('',(#665),#463,.T.);
#4156=ADVANCED_FACE('',(#666),#464,.T.);
#4157=ADVANCED_FACE('',(#667),#465,.T.);
#4158=ADVANCED_FACE('',(#668),#466,.T.);
#4159=ADVANCED_FACE('',(#669),#467,.T.);
#4160=ADVANCED_FACE('',(#670,#325),#468,.T.);
#4161=ADVANCED_FACE('',(#671,#326),#469,.F.);
#4295=CLOSED_SHELL('',(#4115,#4116,#4117,#4118,#4119,#4120,#4121,#4122,
#4123,#4124,#4125,#4126,#4127,#4128,#4129,#4130,#4131,#4132,#4133,#4134,
#4135,#4136,#4137,#4138,#4139,#4140,#4141,#4142,#4143,#4144,#4145,#4146,
#4147,#4148,#4149,#4150,#4151,#4152,#4153,#4154,#4155,#4156,#4157,#4158,
#4159,#4160,#4161));
#4749=AXIS2_PLACEMENT_3D('',#7019,#5490,#5491);
#4750=AXIS2_PLACEMENT_3D('',#7020,#5492,#5493);
#4751=AXIS2_PLACEMENT_3D('',#7029,#5498,#5499);
#4752=AXIS2_PLACEMENT_3D('',#7035,#5503,#5504);
#4753=AXIS2_PLACEMENT_3D('',#7041,#5508,#5509);
#4754=AXIS2_PLACEMENT_3D('',#7047,#5513,#5514);
#4755=AXIS2_PLACEMENT_3D('',#7053,#5518,#5519);
#4756=AXIS2_PLACEMENT_3D('',#7059,#5523,#5524);
#4757=AXIS2_PLACEMENT_3D('',#7065,#5528,#5529);
#4758=AXIS2_PLACEMENT_3D('',#7071,#5533,#5534);
#4759=AXIS2_PLACEMENT_3D('',#7077,#5538,#5539);
#4760=AXIS2_PLACEMENT_3D('',#7086,#5544,#5545);
#4761=AXIS2_PLACEMENT_3D('',#7092,#5549,#5550);
#4762=AXIS2_PLACEMENT_3D('',#7098,#5554,#5555);
#4763=AXIS2_PLACEMENT_3D('',#7104,#5559,#5560);
#4764=AXIS2_PLACEMENT_3D('',#7110,#5564,#5565);
#4765=AXIS2_PLACEMENT_3D('',#7116,#5569,#5570);
#4766=AXIS2_PLACEMENT_3D('',#7122,#5574,#5575);
#4767=AXIS2_PLACEMENT_3D('',#7128,#5579,#5580);
#4768=AXIS2_PLACEMENT_3D('',#7134,#5584,#5585);
#4769=AXIS2_PLACEMENT_3D('',#7143,#5590,#5591);
#4770=AXIS2_PLACEMENT_3D('',#7149,#5595,#5596);
#4771=AXIS2_PLACEMENT_3D('',#7155,#5600,#5601);
#4772=AXIS2_PLACEMENT_3D('',#7161,#5605,#5606);
#4773=AXIS2_PLACEMENT_3D('',#7167,#5610,#5611);
#4774=AXIS2_PLACEMENT_3D('',#7173,#5615,#5616);
#4775=AXIS2_PLACEMENT_3D('',#7179,#5620,#5621);
#4776=AXIS2_PLACEMENT_3D('',#7185,#5625,#5626);
#4777=AXIS2_PLACEMENT_3D('',#7191,#5630,#5631);
#4778=AXIS2_PLACEMENT_3D('',#7200,#5636,#5637);
#4779=AXIS2_PLACEMENT_3D('',#7206,#5641,#5642);
#4780=AXIS2_PLACEMENT_3D('',#7212,#5646,#5647);
#4781=AXIS2_PLACEMENT_3D('',#7218,#5651,#5652);
#4782=AXIS2_PLACEMENT_3D('',#7224,#5656,#5657);
#4783=AXIS2_PLACEMENT_3D('',#7230,#5661,#5662);
#4784=AXIS2_PLACEMENT_3D('',#7236,#5666,#5667);
#4785=AXIS2_PLACEMENT_3D('',#7242,#5671,#5672);
#4786=AXIS2_PLACEMENT_3D('',#7248,#5676,#5677);
#4787=AXIS2_PLACEMENT_3D('',#7250,#5678,#5679);
#4788=AXIS2_PLACEMENT_3D('',#7253,#5681,#5682);
#4789=AXIS2_PLACEMENT_3D('',#7254,#5683,#5684);
#4790=AXIS2_PLACEMENT_3D('',#7260,#5688,#5689);
#4791=AXIS2_PLACEMENT_3D('',#7266,#5693,#5694);
#4792=AXIS2_PLACEMENT_3D('',#7269,#5697,#5698);
#4793=AXIS2_PLACEMENT_3D('',#7275,#5702,#5703);
#4794=AXIS2_PLACEMENT_3D('',#7278,#5706,#5707);
#4795=AXIS2_PLACEMENT_3D('',#7284,#5711,#5712);
#4796=AXIS2_PLACEMENT_3D('',#7287,#5715,#5716);
#4797=AXIS2_PLACEMENT_3D('',#7290,#5719,#5720);
#4798=AXIS2_PLACEMENT_3D('',#7291,#5721,#5722);
#5490=DIRECTION('axis',(0.,0.,1.));
#5491=DIRECTION('refdir',(1.,0.,0.));
#5492=DIRECTION('center_axis',(0.,0.,-1.));
#5493=DIRECTION('ref_axis',(0.,1.,0.));
#5494=DIRECTION('',(0.,1.,0.));
#5495=DIRECTION('',(1.,0.,0.));
#5496=DIRECTION('',(0.,-1.,0.));
#5497=DIRECTION('',(1.,0.,0.));
#5498=DIRECTION('center_axis',(0.,1.,-8.88178419700125E-16));
#5499=DIRECTION('ref_axis',(0.,8.88178419700125E-16,1.));
#5500=DIRECTION('',(0.,8.88178419700125E-16,1.));
#5501=DIRECTION('',(1.,0.,0.));
#5502=DIRECTION('',(0.,-8.88178419700125E-16,-1.));
#5503=DIRECTION('center_axis',(0.,-7.40148683083439E-16,-1.));
#5504=DIRECTION('ref_axis',(0.,1.,-7.40148683083439E-16));
#5505=DIRECTION('',(0.,1.,-7.40148683083439E-16));
#5506=DIRECTION('',(1.,0.,0.));
#5507=DIRECTION('',(0.,-1.,7.40148683083439E-16));
#5508=DIRECTION('center_axis',(0.,-0.707106781186547,-0.707106781186548));
#5509=DIRECTION('ref_axis',(0.,0.707106781186548,-0.707106781186547));
#5510=DIRECTION('',(0.,0.707106781186548,-0.707106781186547));
#5511=DIRECTION('',(1.,0.,0.));
#5512=DIRECTION('',(0.,-0.707106781186548,0.707106781186547));
#5513=DIRECTION('center_axis',(0.,-1.,2.77555756156289E-16));
#5514=DIRECTION('ref_axis',(0.,-2.77555756156289E-16,-1.));
#5515=DIRECTION('',(0.,-2.77555756156289E-16,-1.));
#5516=DIRECTION('',(1.,0.,0.));
#5517=DIRECTION('',(0.,2.77555756156289E-16,1.));
#5518=DIRECTION('center_axis',(0.,-0.707106781186547,0.707106781186548));
#5519=DIRECTION('ref_axis',(0.,-0.707106781186548,-0.707106781186547));
#5520=DIRECTION('',(0.,-0.707106781186548,-0.707106781186547));
#5521=DIRECTION('',(1.,0.,0.));
#5522=DIRECTION('',(0.,0.707106781186548,0.707106781186547));
#5523=DIRECTION('center_axis',(0.,7.40148683083438E-16,1.));
#5524=DIRECTION('ref_axis',(0.,-1.,7.40148683083438E-16));
#5525=DIRECTION('',(0.,-1.,7.40148683083438E-16));
#5526=DIRECTION('',(1.,0.,0.));
#5527=DIRECTION('',(0.,1.,-7.40148683083438E-16));
#5528=DIRECTION('center_axis',(0.,1.,-4.44089209850063E-16));
#5529=DIRECTION('ref_axis',(0.,4.44089209850063E-16,1.));
#5530=DIRECTION('',(0.,4.44089209850063E-16,1.));
#5531=DIRECTION('',(1.,0.,0.));
#5532=DIRECTION('',(0.,-4.44089209850063E-16,-1.));
#5533=DIRECTION('center_axis',(0.,2.41352831440251E-16,1.));
#5534=DIRECTION('ref_axis',(0.,-1.,2.41352831440251E-16));
#5535=DIRECTION('',(0.,-1.,2.41352831440251E-16));
#5536=DIRECTION('',(-1.,0.,0.));
#5537=DIRECTION('',(0.,1.,-2.41352831440251E-16));
#5538=DIRECTION('center_axis',(0.,-1.,2.41352831440251E-16));
#5539=DIRECTION('ref_axis',(0.,-2.41352831440251E-16,-1.));
#5540=DIRECTION('',(0.,-2.41352831440251E-16,-1.));
#5541=DIRECTION('',(1.,0.,0.));
#5542=DIRECTION('',(0.,2.41352831440251E-16,1.));
#5543=DIRECTION('',(1.,0.,0.));
#5544=DIRECTION('center_axis',(0.,0.,-1.));
#5545=DIRECTION('ref_axis',(0.,1.,0.));
#5546=DIRECTION('',(0.,1.,0.));
#5547=DIRECTION('',(1.,0.,0.));
#5548=DIRECTION('',(0.,-1.,0.));
#5549=DIRECTION('center_axis',(0.,-1.,0.));
#5550=DIRECTION('ref_axis',(0.,0.,-1.));
#5551=DIRECTION('',(0.,0.,-1.));
#5552=DIRECTION('',(1.,0.,0.));
#5553=DIRECTION('',(0.,0.,1.));
#5554=DIRECTION('center_axis',(0.,-0.707106781186547,0.707106781186548));
#5555=DIRECTION('ref_axis',(0.,-0.707106781186548,-0.707106781186547));
#5556=DIRECTION('',(0.,-0.707106781186548,-0.707106781186547));
#5557=DIRECTION('',(1.,0.,0.));
#5558=DIRECTION('',(0.,0.707106781186548,0.707106781186547));
#5559=DIRECTION('center_axis',(0.,0.,1.));
#5560=DIRECTION('ref_axis',(0.,-1.,0.));
#5561=DIRECTION('',(0.,-1.,0.));
#5562=DIRECTION('',(1.,0.,0.));
#5563=DIRECTION('',(0.,1.,0.));
#5564=DIRECTION('center_axis',(0.,0.707106781186548,0.707106781186547));
#5565=DIRECTION('ref_axis',(0.,-0.707106781186547,0.707106781186548));
#5566=DIRECTION('',(0.,-0.707106781186547,0.707106781186548));
#5567=DIRECTION('',(1.,0.,0.));
#5568=DIRECTION('',(0.,0.707106781186547,-0.707106781186548));
#5569=DIRECTION('center_axis',(0.,1.,0.));
#5570=DIRECTION('ref_axis',(0.,0.,1.));
#5571=DIRECTION('',(0.,0.,1.));
#5572=DIRECTION('',(1.,0.,0.));
#5573=DIRECTION('',(0.,0.,-1.));
#5574=DIRECTION('center_axis',(0.,0.,-1.));
#5575=DIRECTION('ref_axis',(0.,1.,0.));
#5576=DIRECTION('',(0.,1.,0.));
#5577=DIRECTION('',(1.,0.,0.));
#5578=DIRECTION('',(0.,-1.,0.));
#5579=DIRECTION('center_axis',(0.,1.,-2.41352831440251E-16));
#5580=DIRECTION('ref_axis',(0.,2.41352831440251E-16,1.));
#5581=DIRECTION('',(0.,2.41352831440251E-16,1.));
#5582=DIRECTION('',(-1.,0.,0.));
#5583=DIRECTION('',(0.,-2.41352831440251E-16,-1.));
#5584=DIRECTION('center_axis',(0.,0.,1.));
#5585=DIRECTION('ref_axis',(0.,-1.,0.));
#5586=DIRECTION('',(0.,-1.,0.));
#5587=DIRECTION('',(1.,0.,0.));
#5588=DIRECTION('',(0.,1.,0.));
#5589=DIRECTION('',(1.,0.,0.));
#5590=DIRECTION('center_axis',(0.,-1.,0.));
#5591=DIRECTION('ref_axis',(0.,0.,-1.));
#5592=DIRECTION('',(0.,0.,-1.));
#5593=DIRECTION('',(1.,0.,0.));
#5594=DIRECTION('',(0.,0.,1.));
#5595=DIRECTION('center_axis',(0.,0.,1.));
#5596=DIRECTION('ref_axis',(0.,-1.,0.));
#5597=DIRECTION('',(0.,-1.,0.));
#5598=DIRECTION('',(1.,0.,0.));
#5599=DIRECTION('',(0.,1.,0.));
#5600=DIRECTION('center_axis',(0.,0.707106781186548,0.707106781186548));
#5601=DIRECTION('ref_axis',(0.,-0.707106781186548,0.707106781186548));
#5602=DIRECTION('',(0.,-0.707106781186548,0.707106781186548));
#5603=DIRECTION('',(1.,0.,0.));
#5604=DIRECTION('',(0.,0.707106781186548,-0.707106781186548));
#5605=DIRECTION('center_axis',(0.,1.,0.));
#5606=DIRECTION('ref_axis',(0.,0.,1.));
#5607=DIRECTION('',(0.,0.,1.));
#5608=DIRECTION('',(1.,0.,0.));
#5609=DIRECTION('',(0.,0.,-1.));
#5610=DIRECTION('center_axis',(0.,0.707106781186548,-0.707106781186547));
#5611=DIRECTION('ref_axis',(0.,0.707106781186547,0.707106781186548));
#5612=DIRECTION('',(0.,0.707106781186547,0.707106781186548));
#5613=DIRECTION('',(1.,0.,0.));
#5614=DIRECTION('',(0.,-0.707106781186547,-0.707106781186548));
#5615=DIRECTION('center_axis',(0.,-7.40148683083438E-16,-1.));
#5616=DIRECTION('ref_axis',(0.,1.,-7.40148683083438E-16));
#5617=DIRECTION('',(0.,1.,-7.40148683083438E-16));
#5618=DIRECTION('',(1.,0.,0.));
#5619=DIRECTION('',(0.,-1.,7.40148683083438E-16));
#5620=DIRECTION('center_axis',(0.,-1.,0.));
#5621=DIRECTION('ref_axis',(0.,0.,-1.));
#5622=DIRECTION('',(0.,0.,-1.));
#5623=DIRECTION('',(1.,0.,0.));
#5624=DIRECTION('',(0.,0.,1.));
#5625=DIRECTION('center_axis',(0.,0.,-1.));
#5626=DIRECTION('ref_axis',(0.,1.,0.));
#5627=DIRECTION('',(0.,1.,0.));
#5628=DIRECTION('',(-1.,0.,0.));
#5629=DIRECTION('',(0.,-1.,0.));
#5630=DIRECTION('center_axis',(0.,1.,0.));
#5631=DIRECTION('ref_axis',(0.,0.,1.));
#5632=DIRECTION('',(0.,0.,1.));
#5633=DIRECTION('',(1.,0.,0.));
#5634=DIRECTION('',(0.,0.,-1.));
#5635=DIRECTION('',(1.,0.,0.));
#5636=DIRECTION('center_axis',(0.,0.,1.));
#5637=DIRECTION('ref_axis',(0.,-1.,0.));
#5638=DIRECTION('',(0.,-1.,0.));
#5639=DIRECTION('',(1.,0.,0.));
#5640=DIRECTION('',(0.,1.,0.));
#5641=DIRECTION('center_axis',(0.,1.,0.));
#5642=DIRECTION('ref_axis',(0.,0.,1.));
#5643=DIRECTION('',(0.,0.,1.));
#5644=DIRECTION('',(1.,0.,0.));
#5645=DIRECTION('',(0.,0.,-1.));
#5646=DIRECTION('center_axis',(0.,0.707106781186547,-0.707106781186548));
#5647=DIRECTION('ref_axis',(0.,0.707106781186548,0.707106781186547));
#5648=DIRECTION('',(0.,0.707106781186548,0.707106781186547));
#5649=DIRECTION('',(1.,0.,0.));
#5650=DIRECTION('',(0.,-0.707106781186548,-0.707106781186547));
#5651=DIRECTION('center_axis',(0.,0.,-1.));
#5652=DIRECTION('ref_axis',(0.,1.,0.));
#5653=DIRECTION('',(0.,1.,0.));
#5654=DIRECTION('',(1.,0.,0.));
#5655=DIRECTION('',(0.,-1.,0.));
#5656=DIRECTION('center_axis',(0.,-0.707106781186547,-0.707106781186548));
#5657=DIRECTION('ref_axis',(0.,0.707106781186548,-0.707106781186547));
#5658=DIRECTION('',(0.,0.707106781186548,-0.707106781186547));
#5659=DIRECTION('',(1.,0.,0.));
#5660=DIRECTION('',(0.,-0.707106781186548,0.707106781186547));
#5661=DIRECTION('center_axis',(0.,-1.,0.));
#5662=DIRECTION('ref_axis',(0.,0.,-1.));
#5663=DIRECTION('',(0.,0.,-1.));
#5664=DIRECTION('',(1.,0.,0.));
#5665=DIRECTION('',(0.,0.,1.));
#5666=DIRECTION('center_axis',(0.,0.,1.));
#5667=DIRECTION('ref_axis',(0.,-1.,0.));
#5668=DIRECTION('',(0.,-1.,0.));
#5669=DIRECTION('',(1.,0.,0.));
#5670=DIRECTION('',(0.,1.,0.));
#5671=DIRECTION('center_axis',(0.,-1.,0.));
#5672=DIRECTION('ref_axis',(0.,0.,-1.));
#5673=DIRECTION('',(0.,0.,-1.));
#5674=DIRECTION('',(-1.,0.,0.));
#5675=DIRECTION('',(0.,0.,1.));
#5676=DIRECTION('center_axis',(1.,0.,0.));
#5677=DIRECTION('ref_axis',(0.,0.,-1.));
#5678=DIRECTION('center_axis',(1.,0.,0.));
#5679=DIRECTION('ref_axis',(0.,0.,-1.));
#5680=DIRECTION('',(1.,0.,0.));
#5681=DIRECTION('center_axis',(-1.,0.,0.));
#5682=DIRECTION('ref_axis',(0.,0.,-1.));
#5683=DIRECTION('center_axis',(0.,1.,0.));
#5684=DIRECTION('ref_axis',(0.,0.,1.));
#5685=DIRECTION('',(0.,0.,1.));
#5686=DIRECTION('',(1.,0.,0.));
#5687=DIRECTION('',(0.,0.,1.));
#5688=DIRECTION('center_axis',(0.,1.,0.));
#5689=DIRECTION('ref_axis',(0.,0.,1.));
#5690=DIRECTION('',(0.,0.,1.));
#5691=DIRECTION('',(1.,0.,0.));
#5692=DIRECTION('',(0.,0.,1.));
#5693=DIRECTION('center_axis',(0.,0.,-1.));
#5694=DIRECTION('ref_axis',(0.,1.,0.));
#5695=DIRECTION('',(0.,1.,0.));
#5696=DIRECTION('',(0.,1.,0.));
#5697=DIRECTION('center_axis',(0.,0.,-1.));
#5698=DIRECTION('ref_axis',(0.,1.,0.));
#5699=DIRECTION('',(0.,1.,0.));
#5700=DIRECTION('',(1.,0.,0.));
#5701=DIRECTION('',(0.,1.,0.));
#5702=DIRECTION('center_axis',(0.,-1.,0.));
#5703=DIRECTION('ref_axis',(0.,0.,-1.));
#5704=DIRECTION('',(0.,0.,-1.));
#5705=DIRECTION('',(0.,0.,-1.));
#5706=DIRECTION('center_axis',(0.,-1.,0.));
#5707=DIRECTION('ref_axis',(0.,0.,-1.));
#5708=DIRECTION('',(0.,0.,-1.));
#5709=DIRECTION('',(1.,0.,0.));
#5710=DIRECTION('',(0.,0.,-1.));
#5711=DIRECTION('center_axis',(0.,0.,1.));
#5712=DIRECTION('ref_axis',(0.,-1.,0.));
#5713=DIRECTION('',(0.,-1.,0.));
#5714=DIRECTION('',(0.,-1.,0.));
#5715=DIRECTION('center_axis',(0.,0.,1.));
#5716=DIRECTION('ref_axis',(0.,-1.,0.));
#5717=DIRECTION('',(0.,-1.,0.));
#5718=DIRECTION('',(0.,-1.,0.));
#5719=DIRECTION('center_axis',(1.,0.,0.));
#5720=DIRECTION('ref_axis',(0.,0.,-1.));
#5721=DIRECTION('center_axis',(1.,0.,0.));
#5722=DIRECTION('ref_axis',(0.,0.,-1.));
#7019=CARTESIAN_POINT('',(0.,0.,0.));
#7020=CARTESIAN_POINT('Origin',(-0.1,0.82,-0.3));
#7021=CARTESIAN_POINT('',(0.,0.82,-0.3));
#7022=CARTESIAN_POINT('',(0.,1.,-0.3));
#7023=CARTESIAN_POINT('',(0.,0.41,-0.3));
#7024=CARTESIAN_POINT('',(20.,0.82,-0.3));
#7025=CARTESIAN_POINT('',(-0.1,0.82,-0.3));
#7026=CARTESIAN_POINT('',(20.,1.,-0.3));
#7027=CARTESIAN_POINT('',(20.,0.41,-0.3));
#7028=CARTESIAN_POINT('',(-0.05,1.,-0.3));
#7029=CARTESIAN_POINT('Origin',(-0.1,0.82,-0.55));
#7030=CARTESIAN_POINT('',(0.,0.82,-0.55));
#7031=CARTESIAN_POINT('',(0.,0.82,-0.275));
#7032=CARTESIAN_POINT('',(20.,0.82,-0.55));
#7033=CARTESIAN_POINT('',(-0.1,0.82,-0.55));
#7034=CARTESIAN_POINT('',(20.,0.82,-0.275));
#7035=CARTESIAN_POINT('Origin',(-0.1,0.67,-0.55));
#7036=CARTESIAN_POINT('',(0.,0.67,-0.55));
#7037=CARTESIAN_POINT('',(0.,0.335,-0.55));
#7038=CARTESIAN_POINT('',(20.,0.67,-0.55));
#7039=CARTESIAN_POINT('',(-0.1,0.67,-0.55));
#7040=CARTESIAN_POINT('',(20.,0.335,-0.55));
#7041=CARTESIAN_POINT('Origin',(-0.1,0.42,-0.3));
#7042=CARTESIAN_POINT('',(0.,0.42,-0.3));
#7043=CARTESIAN_POINT('',(0.,0.24,-0.12));
#7044=CARTESIAN_POINT('',(20.,0.42,-0.3));
#7045=CARTESIAN_POINT('',(-0.1,0.42,-0.3));
#7046=CARTESIAN_POINT('',(20.,0.24,-0.12));
#7047=CARTESIAN_POINT('Origin',(-0.1,0.42,0.3));
#7048=CARTESIAN_POINT('',(0.,0.42,0.3));
#7049=CARTESIAN_POINT('',(0.,0.42,0.15));
#7050=CARTESIAN_POINT('',(20.,0.42,0.3));
#7051=CARTESIAN_POINT('',(-0.1,0.42,0.3));
#7052=CARTESIAN_POINT('',(20.,0.42,0.15));
#7053=CARTESIAN_POINT('Origin',(-0.1,0.67,0.55));
#7054=CARTESIAN_POINT('',(0.,0.67,0.55));
#7055=CARTESIAN_POINT('',(6.93889390390723E-18,0.365,0.245));
#7056=CARTESIAN_POINT('',(20.,0.67,0.55));
#7057=CARTESIAN_POINT('',(-0.1,0.67,0.55));
#7058=CARTESIAN_POINT('',(20.,0.365,0.245));
#7059=CARTESIAN_POINT('Origin',(-0.1,0.82,0.55));
#7060=CARTESIAN_POINT('',(0.,0.82,0.55));
#7061=CARTESIAN_POINT('',(0.,0.41,0.55));
#7062=CARTESIAN_POINT('',(20.,0.82,0.55));
#7063=CARTESIAN_POINT('',(-0.1,0.82,0.55));
#7064=CARTESIAN_POINT('',(20.,0.41,0.55));
#7065=CARTESIAN_POINT('Origin',(-0.1,0.82,0.3));
#7066=CARTESIAN_POINT('',(0.,0.82,0.3));
#7067=CARTESIAN_POINT('',(0.,0.82,0.15));
#7068=CARTESIAN_POINT('',(20.,0.82,0.3));
#7069=CARTESIAN_POINT('',(-0.1,0.82,0.3));
#7070=CARTESIAN_POINT('',(20.,0.82,0.15));
#7071=CARTESIAN_POINT('Origin',(-0.1,1.05,0.3));
#7072=CARTESIAN_POINT('',(0.,1.,0.3));
#7073=CARTESIAN_POINT('',(0.,0.525,0.3));
#7074=CARTESIAN_POINT('',(20.,1.,0.3));
#7075=CARTESIAN_POINT('',(-0.05,1.,0.3));
#7076=CARTESIAN_POINT('',(20.,0.525,0.3));
#7077=CARTESIAN_POINT('Origin',(-0.1,-0.3,-0.82));
#7078=CARTESIAN_POINT('',(0.,-0.3,-0.82));
#7079=CARTESIAN_POINT('',(0.,-0.3,-1.));
#7080=CARTESIAN_POINT('',(0.,-0.3,-0.41));
#7081=CARTESIAN_POINT('',(20.,-0.3,-0.82));
#7082=CARTESIAN_POINT('',(-0.1,-0.3,-0.82));
#7083=CARTESIAN_POINT('',(20.,-0.3,-1.));
#7084=CARTESIAN_POINT('',(20.,-0.3,-0.41));
#7085=CARTESIAN_POINT('',(-0.05,-0.3,-1.));
#7086=CARTESIAN_POINT('Origin',(-0.1,-0.55,-0.82));
#7087=CARTESIAN_POINT('',(0.,-0.55,-0.82));
#7088=CARTESIAN_POINT('',(0.,-0.275,-0.82));
#7089=CARTESIAN_POINT('',(20.,-0.55,-0.82));
#7090=CARTESIAN_POINT('',(-0.1,-0.55,-0.82));
#7091=CARTESIAN_POINT('',(20.,-0.275,-0.82));
#7092=CARTESIAN_POINT('Origin',(-0.1,-0.55,-0.67));
#7093=CARTESIAN_POINT('',(0.,-0.55,-0.67));
#7094=CARTESIAN_POINT('',(0.,-0.55,-0.335));
#7095=CARTESIAN_POINT('',(20.,-0.55,-0.67));
#7096=CARTESIAN_POINT('',(-0.1,-0.55,-0.67));
#7097=CARTESIAN_POINT('',(20.,-0.55,-0.335));
#7098=CARTESIAN_POINT('Origin',(-0.1,-0.3,-0.42));
#7099=CARTESIAN_POINT('',(0.,-0.3,-0.42));
#7100=CARTESIAN_POINT('',(0.,-0.12,-0.24));
#7101=CARTESIAN_POINT('',(20.,-0.3,-0.42));
#7102=CARTESIAN_POINT('',(-0.1,-0.3,-0.42));
#7103=CARTESIAN_POINT('',(20.,-0.12,-0.24));
#7104=CARTESIAN_POINT('Origin',(-0.1,0.3,-0.42));
#7105=CARTESIAN_POINT('',(0.,0.3,-0.42));
#7106=CARTESIAN_POINT('',(0.,0.15,-0.42));
#7107=CARTESIAN_POINT('',(20.,0.3,-0.42));
#7108=CARTESIAN_POINT('',(-0.1,0.3,-0.42));
#7109=CARTESIAN_POINT('',(20.,0.15,-0.42));
#7110=CARTESIAN_POINT('Origin',(-0.1,0.55,-0.67));
#7111=CARTESIAN_POINT('',(0.,0.55,-0.67));
#7112=CARTESIAN_POINT('',(0.,0.245,-0.365));
#7113=CARTESIAN_POINT('',(20.,0.55,-0.67));
#7114=CARTESIAN_POINT('',(-0.1,0.55,-0.67));
#7115=CARTESIAN_POINT('',(20.,0.245,-0.365));
#7116=CARTESIAN_POINT('Origin',(-0.1,0.55,-0.82));
#7117=CARTESIAN_POINT('',(0.,0.55,-0.82));
#7118=CARTESIAN_POINT('',(0.,0.55,-0.41));
#7119=CARTESIAN_POINT('',(20.,0.55,-0.82));
#7120=CARTESIAN_POINT('',(-0.1,0.55,-0.82));
#7121=CARTESIAN_POINT('',(20.,0.55,-0.41));
#7122=CARTESIAN_POINT('Origin',(-0.1,0.3,-0.82));
#7123=CARTESIAN_POINT('',(0.,0.3,-0.82));
#7124=CARTESIAN_POINT('',(0.,0.15,-0.82));
#7125=CARTESIAN_POINT('',(20.,0.3,-0.82));
#7126=CARTESIAN_POINT('',(-0.1,0.3,-0.82));
#7127=CARTESIAN_POINT('',(20.,0.15,-0.82));
#7128=CARTESIAN_POINT('Origin',(-0.1,0.3,-1.05));
#7129=CARTESIAN_POINT('',(0.,0.3,-1.));
#7130=CARTESIAN_POINT('',(0.,0.3,-0.525));
#7131=CARTESIAN_POINT('',(20.,0.3,-1.));
#7132=CARTESIAN_POINT('',(-0.05,0.3,-1.));
#7133=CARTESIAN_POINT('',(20.,0.3,-0.525));
#7134=CARTESIAN_POINT('Origin',(-0.1,-0.82,0.3));
#7135=CARTESIAN_POINT('',(0.,-0.82,0.3));
#7136=CARTESIAN_POINT('',(0.,-1.,0.3));
#7137=CARTESIAN_POINT('',(0.,-0.41,0.3));
#7138=CARTESIAN_POINT('',(20.,-0.82,0.3));
#7139=CARTESIAN_POINT('',(-0.1,-0.82,0.3));
#7140=CARTESIAN_POINT('',(20.,-1.,0.3));
#7141=CARTESIAN_POINT('',(20.,-0.41,0.3));
#7142=CARTESIAN_POINT('',(-0.05,-1.,0.3));
#7143=CARTESIAN_POINT('Origin',(-0.1,-0.82,0.55));
#7144=CARTESIAN_POINT('',(0.,-0.82,0.55));
#7145=CARTESIAN_POINT('',(0.,-0.82,0.275));
#7146=CARTESIAN_POINT('',(20.,-0.82,0.55));
#7147=CARTESIAN_POINT('',(-0.1,-0.82,0.55));
#7148=CARTESIAN_POINT('',(20.,-0.82,0.275));
#7149=CARTESIAN_POINT('Origin',(-0.1,-0.67,0.55));
#7150=CARTESIAN_POINT('',(0.,-0.67,0.55));
#7151=CARTESIAN_POINT('',(0.,-0.335,0.55));
#7152=CARTESIAN_POINT('',(20.,-0.67,0.55));
#7153=CARTESIAN_POINT('',(-0.1,-0.67,0.55));
#7154=CARTESIAN_POINT('',(20.,-0.335,0.55));
#7155=CARTESIAN_POINT('Origin',(-0.1,-0.42,0.3));
#7156=CARTESIAN_POINT('',(0.,-0.42,0.3));
#7157=CARTESIAN_POINT('',(-6.93889390390723E-18,-0.24,0.12));
#7158=CARTESIAN_POINT('',(20.,-0.42,0.3));
#7159=CARTESIAN_POINT('',(-0.1,-0.42,0.3));
#7160=CARTESIAN_POINT('',(20.,-0.24,0.12));
#7161=CARTESIAN_POINT('Origin',(-0.1,-0.42,-0.3));
#7162=CARTESIAN_POINT('',(0.,-0.42,-0.3));
#7163=CARTESIAN_POINT('',(0.,-0.42,-0.15));
#7164=CARTESIAN_POINT('',(20.,-0.42,-0.3));
#7165=CARTESIAN_POINT('',(-0.1,-0.42,-0.3));
#7166=CARTESIAN_POINT('',(20.,-0.42,-0.15));
#7167=CARTESIAN_POINT('Origin',(-0.1,-0.67,-0.55));
#7168=CARTESIAN_POINT('',(0.,-0.67,-0.55));
#7169=CARTESIAN_POINT('',(0.,-0.365,-0.245));
#7170=CARTESIAN_POINT('',(20.,-0.67,-0.55));
#7171=CARTESIAN_POINT('',(-0.1,-0.67,-0.55));
#7172=CARTESIAN_POINT('',(20.,-0.365,-0.245));
#7173=CARTESIAN_POINT('Origin',(-0.1,-0.82,-0.55));
#7174=CARTESIAN_POINT('',(0.,-0.82,-0.55));
#7175=CARTESIAN_POINT('',(0.,-0.41,-0.55));
#7176=CARTESIAN_POINT('',(20.,-0.82,-0.55));
#7177=CARTESIAN_POINT('',(-0.1,-0.82,-0.55));
#7178=CARTESIAN_POINT('',(20.,-0.41,-0.55));
#7179=CARTESIAN_POINT('Origin',(-0.1,-0.82,-0.3));
#7180=CARTESIAN_POINT('',(0.,-0.82,-0.3));
#7181=CARTESIAN_POINT('',(0.,-0.82,-0.15));
#7182=CARTESIAN_POINT('',(20.,-0.82,-0.3));
#7183=CARTESIAN_POINT('',(-0.1,-0.82,-0.3));
#7184=CARTESIAN_POINT('',(20.,-0.82,-0.15));
#7185=CARTESIAN_POINT('Origin',(-0.1,-1.05,-0.3));
#7186=CARTESIAN_POINT('',(0.,-1.,-0.3));
#7187=CARTESIAN_POINT('',(0.,-0.525,-0.3));
#7188=CARTESIAN_POINT('',(20.,-1.,-0.3));
#7189=CARTESIAN_POINT('',(-0.05,-1.,-0.3));
#7190=CARTESIAN_POINT('',(20.,-0.525,-0.3));
#7191=CARTESIAN_POINT('Origin',(-0.1,0.3,0.82));
#7192=CARTESIAN_POINT('',(0.,0.3,0.82));
#7193=CARTESIAN_POINT('',(0.,0.3,1.));
#7194=CARTESIAN_POINT('',(0.,0.3,0.41));
#7195=CARTESIAN_POINT('',(20.,0.3,0.82));
#7196=CARTESIAN_POINT('',(-0.1,0.3,0.82));
#7197=CARTESIAN_POINT('',(20.,0.3,1.));
#7198=CARTESIAN_POINT('',(20.,0.3,0.41));
#7199=CARTESIAN_POINT('',(-0.05,0.3,1.));
#7200=CARTESIAN_POINT('Origin',(-0.1,0.55,0.82));
#7201=CARTESIAN_POINT('',(0.,0.55,0.82));
#7202=CARTESIAN_POINT('',(0.,0.275,0.82));
#7203=CARTESIAN_POINT('',(20.,0.55,0.82));
#7204=CARTESIAN_POINT('',(-0.1,0.55,0.82));
#7205=CARTESIAN_POINT('',(20.,0.275,0.82));
#7206=CARTESIAN_POINT('Origin',(-0.1,0.55,0.67));
#7207=CARTESIAN_POINT('',(0.,0.55,0.67));
#7208=CARTESIAN_POINT('',(0.,0.55,0.335));
#7209=CARTESIAN_POINT('',(20.,0.55,0.67));
#7210=CARTESIAN_POINT('',(-0.1,0.55,0.67));
#7211=CARTESIAN_POINT('',(20.,0.55,0.335));
#7212=CARTESIAN_POINT('Origin',(-0.1,0.3,0.42));
#7213=CARTESIAN_POINT('',(0.,0.3,0.42));
#7214=CARTESIAN_POINT('',(6.93889390390723E-18,0.12,0.24));
#7215=CARTESIAN_POINT('',(20.,0.3,0.42));
#7216=CARTESIAN_POINT('',(-0.1,0.3,0.42));
#7217=CARTESIAN_POINT('',(20.,0.12,0.24));
#7218=CARTESIAN_POINT('Origin',(-0.1,-0.3,0.42));
#7219=CARTESIAN_POINT('',(0.,-0.3,0.42));
#7220=CARTESIAN_POINT('',(0.,-0.15,0.42));
#7221=CARTESIAN_POINT('',(20.,-0.3,0.42));
#7222=CARTESIAN_POINT('',(-0.1,-0.3,0.42));
#7223=CARTESIAN_POINT('',(20.,-0.15,0.42));
#7224=CARTESIAN_POINT('Origin',(-0.1,-0.55,0.67));
#7225=CARTESIAN_POINT('',(0.,-0.55,0.67));
#7226=CARTESIAN_POINT('',(6.93889390390723E-18,-0.245,0.365));
#7227=CARTESIAN_POINT('',(20.,-0.55,0.67));
#7228=CARTESIAN_POINT('',(-0.1,-0.55,0.67));
#7229=CARTESIAN_POINT('',(20.,-0.245,0.365));
#7230=CARTESIAN_POINT('Origin',(-0.1,-0.55,0.82));
#7231=CARTESIAN_POINT('',(0.,-0.55,0.82));
#7232=CARTESIAN_POINT('',(0.,-0.55,0.41));
#7233=CARTESIAN_POINT('',(20.,-0.55,0.82));
#7234=CARTESIAN_POINT('',(-0.1,-0.55,0.82));
#7235=CARTESIAN_POINT('',(20.,-0.55,0.41));
#7236=CARTESIAN_POINT('Origin',(-0.1,-0.3,0.82));
#7237=CARTESIAN_POINT('',(0.,-0.3,0.82));
#7238=CARTESIAN_POINT('',(0.,-0.15,0.82));
#7239=CARTESIAN_POINT('',(20.,-0.3,0.82));
#7240=CARTESIAN_POINT('',(-0.1,-0.3,0.82));
#7241=CARTESIAN_POINT('',(20.,-0.15,0.82));
#7242=CARTESIAN_POINT('Origin',(-0.1,-0.3,1.05));
#7243=CARTESIAN_POINT('',(0.,-0.3,1.));
#7244=CARTESIAN_POINT('',(0.,-0.3,0.525));
#7245=CARTESIAN_POINT('',(20.,-0.3,1.));
#7246=CARTESIAN_POINT('',(-0.05,-0.3,1.));
#7247=CARTESIAN_POINT('',(20.,-0.3,0.525));
#7248=CARTESIAN_POINT('Origin',(-0.1,0.,0.));
#7249=CARTESIAN_POINT('',(0.,-2.57175827820944E-17,0.21));
#7250=CARTESIAN_POINT('Origin',(0.,0.,0.));
#7251=CARTESIAN_POINT('',(20.,2.57175827820944E-17,0.21));
#7252=CARTESIAN_POINT('',(-0.1,-2.57175827820944E-17,0.21));
#7253=CARTESIAN_POINT('Origin',(20.,0.,0.));
#7254=CARTESIAN_POINT('Origin',(0.,1.,-1.));
#7255=CARTESIAN_POINT('',(0.,1.,1.));
#7256=CARTESIAN_POINT('',(0.,1.,-1.));
#7257=CARTESIAN_POINT('',(20.,1.,1.));
#7258=CARTESIAN_POINT('',(0.,1.,1.));
#7259=CARTESIAN_POINT('',(20.,1.,-1.));
#7260=CARTESIAN_POINT('Origin',(0.,1.,-1.));
#7261=CARTESIAN_POINT('',(20.,1.,-1.));
#7262=CARTESIAN_POINT('',(20.,1.,-1.));
#7263=CARTESIAN_POINT('',(0.,1.,-1.));
#7264=CARTESIAN_POINT('',(0.,1.,-1.));
#7265=CARTESIAN_POINT('',(0.,1.,-1.));
#7266=CARTESIAN_POINT('Origin',(0.,-1.,-1.));
#7267=CARTESIAN_POINT('',(0.,-1.,-1.));
#7268=CARTESIAN_POINT('',(20.,-1.,-1.));
#7269=CARTESIAN_POINT('Origin',(0.,-1.,-1.));
#7270=CARTESIAN_POINT('',(20.,-1.,-1.));
#7271=CARTESIAN_POINT('',(20.,-1.,-1.));
#7272=CARTESIAN_POINT('',(0.,-1.,-1.));
#7273=CARTESIAN_POINT('',(0.,-1.,-1.));
#7274=CARTESIAN_POINT('',(0.,-1.,-1.));
#7275=CARTESIAN_POINT('Origin',(0.,-1.,1.));
#7276=CARTESIAN_POINT('',(0.,-1.,1.));
#7277=CARTESIAN_POINT('',(20.,-1.,1.));
#7278=CARTESIAN_POINT('Origin',(0.,-1.,1.));
#7279=CARTESIAN_POINT('',(20.,-1.,1.));
#7280=CARTESIAN_POINT('',(20.,-1.,1.));
#7281=CARTESIAN_POINT('',(0.,-1.,1.));
#7282=CARTESIAN_POINT('',(0.,-1.,1.));
#7283=CARTESIAN_POINT('',(0.,-1.,1.));
#7284=CARTESIAN_POINT('Origin',(0.,1.,1.));
#7285=CARTESIAN_POINT('',(0.,1.,1.));
#7286=CARTESIAN_POINT('',(20.,1.,1.));
#7287=CARTESIAN_POINT('Origin',(0.,1.,1.));
#7288=CARTESIAN_POINT('',(20.,1.,1.));
#7289=CARTESIAN_POINT('',(0.,1.,1.));
#7290=CARTESIAN_POINT('Origin',(20.,0.,0.));
#7291=CARTESIAN_POINT('Origin',(0.,0.,0.));
#7845=UNCERTAINTY_MEASURE_WITH_UNIT(LENGTH_MEASURE(0.001),#7898,
'DISTANCE_ACCURACY_VALUE',
'Maximum model space distance between geometric entities at asserted c
onnectivities');
#7865=UNCERTAINTY_MEASURE_WITH_UNIT(LENGTH_MEASURE(0.001),#7898,
'DISTANCE_ACCURACY_VALUE',
'Maximum model space distance between geometric entities at asserted c
onnectivities');
#7877=(
GEOMETRIC_REPRESENTATION_CONTEXT(3)
GLOBAL_UNCERTAINTY_ASSIGNED_CONTEXT((#7845))
GLOBAL_UNIT_ASSIGNED_CONTEXT((#7898,#7900,#7901))
REPRESENTATION_CONTEXT('','3D')
);
#7897=(
GEOMETRIC_REPRESENTATION_CONTEXT(3)
GLOBAL_UNCERTAINTY_ASSIGNED_CONTEXT((#7865))
GLOBAL_UNIT_ASSIGNED_CONTEXT((#7898,#7900,#7901))
REPRESENTATION_CONTEXT('','3D')
);
#7898=(
LENGTH_UNIT()
NAMED_UNIT(*)
SI_UNIT(.CENTI.,.METRE.)
);
#7900=(
NAMED_UNIT(*)
PLANE_ANGLE_UNIT()
SI_UNIT($,.RADIAN.)
);
#7901=(
NAMED_UNIT(*)
SI_UNIT($,.STERADIAN.)
SOLID_ANGLE_UNIT()
);
#7913=SHAPE_DEFINITION_REPRESENTATION(#7944,#8010);
#7944=PRODUCT_DEFINITION_SHAPE('',$,#8042);
#8010=SHAPE_REPRESENTATION('',(#4749),#7877);
#8030=PRODUCT_DEFINITION_CONTEXT('part definition',#8125,'design');
#8042=PRODUCT_DEFINITION('Slotted Extrusion - 20 x 20 x 200 mm',
'Slotted Extrusion - 20 x 20 x 200 mm',#8073,#8030);
#8073=PRODUCT_DEFINITION_FORMATION('',$,#8138);
#8125=APPLICATION_CONTEXT(
'Core Data for Automotive Mechanical Design Process');
#8126=PRODUCT_CONTEXT('part definition',#8125,'mechanical');
#8138=PRODUCT('Slotted Extrusion - 20 x 20 x 200 mm',
'Slotted Extrusion - 20 x 20 x 200 mm',
'Slotted Extrusion - 20 x 20 x 200 mm',(#8126));
#8228=COLOUR_RGB('Off White',0.89,0.88,0.83);
#8229=FILL_AREA_STYLE_COLOUR('',#8228);
#8230=FILL_AREA_STYLE('',(#8229));
#8231=SURFACE_STYLE_FILL_AREA(#8230);
#8232=SURFACE_SIDE_STYLE('',(#8231));
#8233=SURFACE_STYLE_USAGE(.BOTH.,#8232);
#8234=PRESENTATION_STYLE_ASSIGNMENT((#8233));
ENDSEC;
END-ISO-10303-21;
